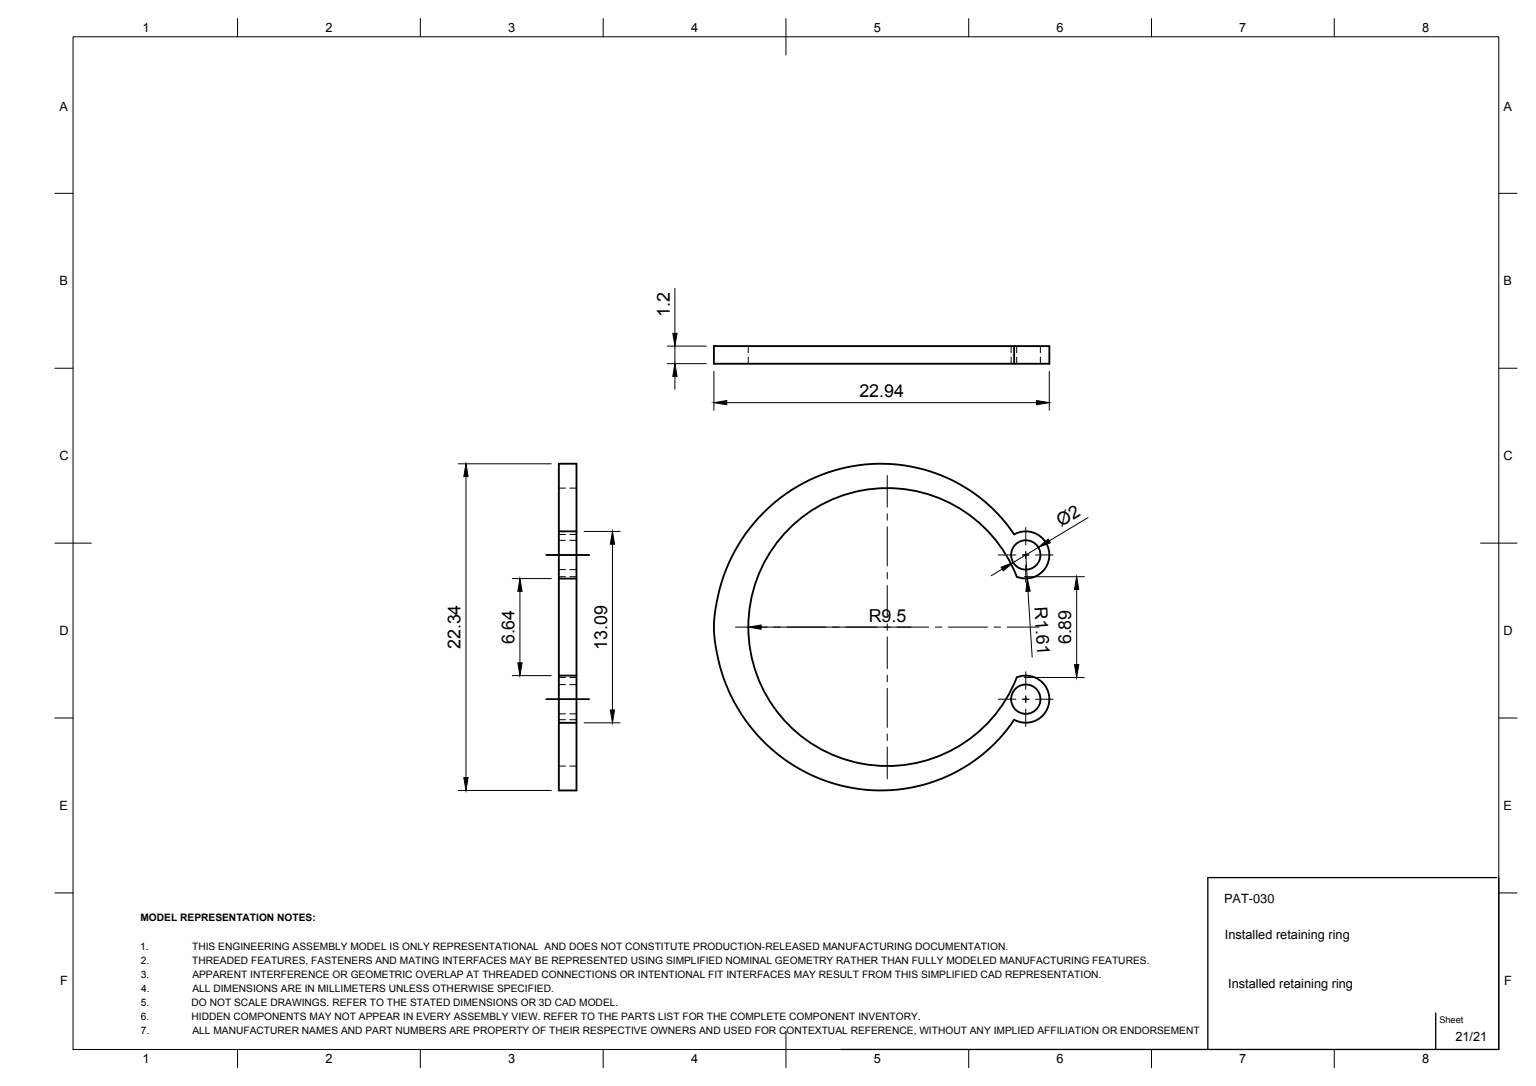
ISO-10303-21;
HEADER;
/* Generated by software containing ST-Developer
 * from STEP Tools, Inc. (www.steptools.com) 
 */

FILE_DESCRIPTION(
/* description */ ('Double-bearing flanged cartridge'),
/* implementation_level */ '2;1');

FILE_NAME(
/* name */ 'Installed retaining ring.step',
/* time_stamp */ '2026-10-28T03:26:40-07:00',
/* author */ (''),
/* organization */ (''),
/* preprocessor_version */ 'ST-DEVELOPER v20.2',
/* originating_system */ 'Autodesk Translation Framework v15.17.0.0',
/* authorisation */ '');

FILE_SCHEMA (('AUTOMOTIVE_DESIGN { 1 0 10303 214 3 1 1 }'));
ENDSEC;

DATA;
#10=MECHANICAL_DESIGN_GEOMETRIC_PRESENTATION_REPRESENTATION('',(#211),#5535);
#11=(
BOUNDED_SURFACE()
B_SPLINE_SURFACE(5,1,((#4887,#4888),(#4889,#4890),(#4891,#4892),(#4893,
#4894),(#4895,#4896),(#4897,#4898),(#4899,#4900),(#4901,#4902),(#4903,#4904),
(#4905,#4906),(#4907,#4908),(#4909,#4910),(#4911,#4912),(#4913,#4914),(#4915,
#4916),(#4917,#4918),(#4919,#4920),(#4921,#4922),(#4923,#4924),(#4925,#4926),
(#4927,#4928),(#4929,#4930),(#4931,#4932),(#4933,#4934),(#4935,#4936),(#4937,
#4938),(#4939,#4940),(#4941,#4942),(#4943,#4944),(#4945,#4946),(#4947,#4948),
(#4949,#4950),(#4951,#4952),(#4953,#4954),(#4955,#4956),(#4957,#4958),(#4959,
#4960),(#4961,#4962),(#4963,#4964),(#4965,#4966),(#4967,#4968),(#4969,#4970),
(#4971,#4972),(#4973,#4974),(#4975,#4976),(#4977,#4978),(#4979,#4980),(#4981,
#4982),(#4983,#4984),(#4985,#4986),(#4987,#4988),(#4989,#4990),(#4991,#4992),
(#4993,#4994),(#4995,#4996),(#4997,#4998),(#4999,#5000),(#5001,#5002),(#5003,
#5004),(#5005,#5006),(#5007,#5008),(#5009,#5010),(#5011,#5012),(#5013,#5014),
(#5015,#5016),(#5017,#5018),(#5019,#5020),(#5021,#5022),(#5023,#5024),(#5025,
#5026),(#5027,#5028),(#5029,#5030),(#5031,#5032),(#5033,#5034),(#5035,#5036),
(#5037,#5038),(#5039,#5040),(#5041,#5042),(#5043,#5044),(#5045,#5046),(#5047,
#5048),(#5049,#5050),(#5051,#5052),(#5053,#5054),(#5055,#5056),(#5057,#5058),
(#5059,#5060),(#5061,#5062),(#5063,#5064),(#5065,#5066),(#5067,#5068),(#5069,
#5070),(#5071,#5072),(#5073,#5074),(#5075,#5076),(#5077,#5078),(#5079,#5080),
(#5081,#5082),(#5083,#5084),(#5085,#5086),(#5087,#5088),(#5089,#5090),(#5091,
#5092),(#5093,#5094),(#5095,#5096),(#5097,#5098),(#5099,#5100),(#5101,#5102),
(#5103,#5104),(#5105,#5106),(#5107,#5108),(#5109,#5110),(#5111,#5112),(#5113,
#5114),(#5115,#5116),(#5117,#5118),(#5119,#5120),(#5121,#5122),(#5123,#5124),
(#5125,#5126),(#5127,#5128),(#5129,#5130),(#5131,#5132),(#5133,#5134),(#5135,
#5136),(#5137,#5138),(#5139,#5140),(#5141,#5142),(#5143,#5144),(#5145,#5146),
(#5147,#5148),(#5149,#5150),(#5151,#5152),(#5153,#5154),(#5155,#5156),(#5157,
#5158),(#5159,#5160),(#5161,#5162),(#5163,#5164),(#5165,#5166),(#5167,#5168),
(#5169,#5170),(#5171,#5172),(#5173,#5174),(#5175,#5176),(#5177,#5178),(#5179,
#5180),(#5181,#5182),(#5183,#5184),(#5185,#5186),(#5187,#5188),(#5189,#5190),
(#5191,#5192),(#5193,#5194),(#5195,#5196),(#5197,#5198),(#5199,#5200),(#5201,
#5202),(#5203,#5204),(#5205,#5206),(#5207,#5208),(#5209,#5210),(#5211,#5212),
(#5213,#5214),(#5215,#5216),(#5217,#5218),(#5219,#5220),(#5221,#5222),(#5223,
#5224),(#5225,#5226),(#5227,#5228),(#5229,#5230),(#5231,#5232),(#5233,#5234),
(#5235,#5236),(#5237,#5238),(#5239,#5240),(#5241,#5242),(#5243,#5244),(#5245,
#5246),(#5247,#5248),(#5249,#5250),(#5251,#5252),(#5253,#5254),(#5255,#5256),
(#5257,#5258),(#5259,#5260),(#5261,#5262),(#5263,#5264),(#5265,#5266),(#5267,
#5268),(#5269,#5270),(#5271,#5272),(#5273,#5274),(#5275,#5276),(#5277,#5278),
(#5279,#5280),(#5281,#5282),(#5283,#5284),(#5285,#5286),(#5287,#5288),(#5289,
#5290),(#5291,#5292),(#5293,#5294),(#5295,#5296)),.UNSPECIFIED.,.F.,.F.,
 .F.)
B_SPLINE_SURFACE_WITH_KNOTS((6,1,1,1,1,1,1,1,1,1,1,1,1,1,1,1,1,1,1,1,1,
1,1,1,1,1,1,1,1,1,1,1,1,1,1,1,1,1,1,1,1,1,1,1,1,1,1,1,1,1,1,1,1,1,1,1,1,
1,1,1,1,1,1,1,1,1,1,1,1,1,1,1,1,1,1,1,1,1,1,1,1,1,1,1,1,1,1,1,1,1,1,1,1,
1,1,1,1,1,1,1,1,1,1,1,1,1,1,1,1,1,1,1,1,1,1,1,1,1,1,1,1,1,1,1,1,1,1,1,1,
1,1,1,1,1,1,1,1,1,1,1,1,1,1,1,1,1,1,1,1,1,1,1,1,1,1,1,1,1,1,1,1,1,1,1,1,
1,1,1,1,1,1,1,1,1,1,1,1,1,1,1,1,1,1,1,1,1,1,1,1,1,1,1,1,1,1,1,1,1,1,1,6),
(2,2),(0.,0.005,0.01,0.015,0.02,0.025,0.03,0.035,0.04,0.045,0.05,0.055,
0.06,0.065,0.07,0.075,0.08,0.085,0.09,0.095,0.1,0.105,0.11,0.115,0.12,0.125,
0.13,0.135,0.14,0.145,0.15,0.155,0.16,0.165,0.17,0.175,0.18,0.185,0.19,
0.195,0.2,0.205,0.21,0.215,0.22,0.225,0.23,0.235,0.24,0.245,0.25,0.255,
0.26,0.265,0.27,0.275,0.28,0.285,0.29,0.295,0.3,0.305,0.31,0.315,0.32,0.325,
0.33,0.335,0.34,0.345,0.35,0.355,0.36,0.365,0.37,0.375,0.38,0.385,0.39,
0.395,0.4,0.405,0.41,0.415,0.42,0.425,0.43,0.435,0.44,0.445,0.45,0.455,
0.46,0.465,0.47,0.475,0.48,0.485,0.49,0.495,0.5,0.505,0.51,0.515,0.52,0.525,
0.53,0.535,0.54,0.545,0.55,0.555,0.56,0.565,0.57,0.575,0.58,0.585,0.59,
0.595,0.6,0.605,0.61,0.615,0.62,0.625,0.63,0.635,0.64,0.645,0.65,0.655,
0.66,0.665,0.67,0.675,0.68,0.685,0.690000000000001,0.695000000000001,0.700000000000001,
0.705000000000001,0.710000000000001,0.715000000000001,0.720000000000001,
0.725000000000001,0.730000000000001,0.735000000000001,0.740000000000001,
0.745000000000001,0.750000000000001,0.755000000000001,0.760000000000001,
0.765000000000001,0.770000000000001,0.775000000000001,0.780000000000001,
0.785000000000001,0.790000000000001,0.795000000000001,0.800000000000001,
0.805000000000001,0.810000000000001,0.815000000000001,0.820000000000001,
0.825000000000001,0.830000000000001,0.835000000000001,0.840000000000001,
0.845000000000001,0.850000000000001,0.855000000000001,0.860000000000001,
0.865000000000001,0.870000000000001,0.875000000000001,0.880000000000001,
0.885000000000001,0.890000000000001,0.895000000000001,0.900000000000001,
0.905000000000001,0.910000000000001,0.915000000000001,0.920000000000001,
0.925000000000001,0.930000000000001,0.935000000000001,0.940000000000001,
0.945000000000001,0.950000000000001,0.955000000000001,0.960000000000001,
0.965000000000001,0.970000000000001,0.975000000000001,0.980000000000001,
0.985000000000001,0.990000000000001,0.995000000000001,1.),(0.,0.12),
 .UNSPECIFIED.)
GEOMETRIC_REPRESENTATION_ITEM()
RATIONAL_B_SPLINE_SURFACE(((1.,1.),(1.,1.),(1.,1.),(1.,1.),(1.,1.),(1.,
1.),(1.,1.),(1.,1.),(1.,1.),(1.,1.),(1.,1.),(1.,1.),(1.,1.),(1.,1.),(1.,
1.),(1.,1.),(1.,1.),(1.,1.),(1.,1.),(1.,1.),(1.,1.),(1.,1.),(1.,1.),(1.,
1.),(1.,1.),(1.,1.),(1.,1.),(1.,1.),(1.,1.),(1.,1.),(1.,1.),(1.,1.),(1.,
1.),(1.,1.),(1.,1.),(1.,1.),(1.,1.),(1.,1.),(1.,1.),(1.,1.),(1.,1.),(1.,
1.),(1.,1.),(1.,1.),(1.,1.),(1.,1.),(1.,1.),(1.,1.),(1.,1.),(1.,1.),(1.,
1.),(1.,1.),(1.,1.),(1.,1.),(1.,1.),(1.,1.),(1.,1.),(1.,1.),(1.,1.),(1.,
1.),(1.,1.),(1.,1.),(1.,1.),(1.,1.),(1.,1.),(1.,1.),(1.,1.),(1.,1.),(1.,
1.),(1.,1.),(1.,1.),(1.,1.),(1.,1.),(1.,1.),(1.,1.),(1.,1.),(1.,1.),(1.,
1.),(1.,1.),(1.,1.),(1.,1.),(1.,1.),(1.,1.),(1.,1.),(1.,1.),(1.,1.),(1.,
1.),(1.,1.),(1.,1.),(1.,1.),(1.,1.),(1.,1.),(1.,1.),(1.,1.),(1.,1.),(1.,
1.),(1.,1.),(1.,1.),(1.,1.),(1.,1.),(1.,1.),(1.,1.),(1.,1.),(1.,1.),(1.,
1.),(1.,1.),(1.,1.),(1.,1.),(1.,1.),(1.,1.),(1.,1.),(1.,1.),(1.,1.),(1.,
1.),(1.,1.),(1.,1.),(1.,1.),(1.,1.),(1.,1.),(1.,1.),(1.,1.),(1.,1.),(1.,
1.),(1.,1.),(1.,1.),(1.,1.),(1.,1.),(1.,1.),(1.,1.),(1.,1.),(1.,1.),(1.,
1.),(1.,1.),(1.,1.),(1.,1.),(1.,1.),(1.,1.),(1.,1.),(1.,1.),(1.,1.),(1.,
1.),(1.,1.),(1.,1.),(1.,1.),(1.,1.),(1.,1.),(1.,1.),(1.,1.),(1.,1.),(1.,
1.),(1.,1.),(1.,1.),(1.,1.),(1.,1.),(1.,1.),(1.,1.),(1.,1.),(1.,1.),(1.,
1.),(1.,1.),(1.,1.),(1.,1.),(1.,1.),(1.,1.),(1.,1.),(1.,1.),(1.,1.),(1.,
1.),(1.,1.),(1.,1.),(1.,1.),(1.,1.),(1.,1.),(1.,1.),(1.,1.),(1.,1.),(1.,
1.),(1.,1.),(1.,1.),(1.,1.),(1.,1.),(1.,1.),(1.,1.),(1.,1.),(1.,1.),(1.,
1.),(1.,1.),(1.,1.),(1.,1.),(1.,1.),(1.,1.),(1.,1.),(1.,1.),(1.,1.),(1.,
1.),(1.,1.),(1.,1.),(1.,1.),(1.,1.),(1.,1.),(1.,1.),(1.,1.),(1.,1.),(1.,
1.),(1.,1.)))
REPRESENTATION_ITEM('')
SURFACE()
);
#12=(
BOUNDED_CURVE()
B_SPLINE_CURVE(5,(#4671,#4672,#4673,#4674,#4675,#4676,#4677,#4678,#4679,
#4680,#4681,#4682,#4683,#4684,#4685,#4686,#4687,#4688,#4689,#4690,#4691,
#4692,#4693,#4694,#4695,#4696,#4697,#4698,#4699,#4700,#4701,#4702,#4703,
#4704,#4705,#4706,#4707,#4708,#4709,#4710,#4711,#4712,#4713,#4714,#4715,
#4716,#4717,#4718,#4719,#4720,#4721,#4722,#4723,#4724,#4725,#4726,#4727,
#4728,#4729,#4730,#4731,#4732,#4733,#4734,#4735,#4736,#4737,#4738,#4739,
#4740,#4741,#4742,#4743,#4744,#4745,#4746,#4747,#4748,#4749,#4750,#4751,
#4752,#4753,#4754,#4755,#4756,#4757,#4758,#4759,#4760,#4761,#4762,#4763,
#4764,#4765,#4766,#4767,#4768,#4769,#4770,#4771,#4772,#4773,#4774,#4775,
#4776,#4777,#4778,#4779,#4780,#4781,#4782,#4783,#4784,#4785,#4786,#4787,
#4788,#4789,#4790,#4791,#4792,#4793,#4794,#4795,#4796,#4797,#4798,#4799,
#4800,#4801,#4802,#4803,#4804,#4805,#4806,#4807,#4808,#4809,#4810,#4811,
#4812,#4813,#4814,#4815,#4816,#4817,#4818,#4819,#4820,#4821,#4822,#4823,
#4824,#4825,#4826,#4827,#4828,#4829,#4830,#4831,#4832,#4833,#4834,#4835,
#4836,#4837,#4838,#4839,#4840,#4841,#4842,#4843,#4844,#4845,#4846,#4847,
#4848,#4849,#4850,#4851,#4852,#4853,#4854,#4855,#4856,#4857,#4858,#4859,
#4860,#4861,#4862,#4863,#4864,#4865),.UNSPECIFIED.,.F.,.F.)
B_SPLINE_CURVE_WITH_KNOTS((6,1,1,1,1,1,1,1,1,1,1,1,1,1,1,1,1,1,1,1,1,1,
1,1,1,1,1,1,1,1,1,1,1,1,1,1,1,1,1,1,1,1,1,1,1,1,1,1,1,1,1,1,1,1,1,1,1,1,
1,1,1,1,1,1,1,1,1,1,1,1,1,1,1,1,1,1,1,1,1,1,1,1,1,1,1,1,1,1,1,1,1,1,1,1,
1,1,1,1,1,1,1,1,1,1,1,1,1,1,1,1,1,1,1,1,1,1,1,1,1,1,1,1,1,1,1,1,1,1,1,1,
1,1,1,1,1,1,1,1,1,1,1,1,1,1,1,1,1,1,1,1,1,1,1,1,1,1,1,1,1,1,1,1,1,1,1,1,
1,1,1,1,1,1,1,1,1,1,1,1,1,1,1,1,1,1,1,1,1,1,1,1,6),(0.02759962388435,0.03,
0.035,0.04,0.045,0.05,0.055,0.06,0.065,0.07,0.075,0.08,0.085,0.09,0.095,
0.1,0.105,0.11,0.115,0.12,0.125,0.13,0.135,0.14,0.145,0.15,0.155,0.16,0.165,
0.17,0.175,0.18,0.185,0.19,0.195,0.2,0.205,0.21,0.215,0.22,0.225,0.23,0.235,
0.24,0.245,0.25,0.255,0.26,0.265,0.27,0.275,0.28,0.285,0.29,0.295,0.3,0.305,
0.31,0.315,0.32,0.325,0.33,0.335,0.34,0.345,0.35,0.355,0.36,0.365,0.37,
0.375,0.38,0.385,0.39,0.395,0.4,0.405,0.41,0.415,0.42,0.425,0.43,0.435,
0.44,0.445,0.45,0.455,0.46,0.465,0.47,0.475,0.48,0.485,0.49,0.495,0.5,0.505,
0.51,0.515,0.52,0.525,0.53,0.535,0.54,0.545,0.55,0.555,0.56,0.565,0.57,
0.575,0.58,0.585,0.59,0.595,0.6,0.605,0.61,0.615,0.62,0.625,0.63,0.635,
0.64,0.645,0.65,0.655,0.66,0.665,0.67,0.675,0.68,0.685,0.690000000000001,
0.695000000000001,0.700000000000001,0.705000000000001,0.710000000000001,
0.715000000000001,0.720000000000001,0.725000000000001,0.730000000000001,
0.735000000000001,0.740000000000001,0.745000000000001,0.750000000000001,
0.755000000000001,0.760000000000001,0.765000000000001,0.770000000000001,
0.775000000000001,0.780000000000001,0.785000000000001,0.790000000000001,
0.795000000000001,0.800000000000001,0.805000000000001,0.810000000000001,
0.815000000000001,0.820000000000001,0.825000000000001,0.830000000000001,
0.835000000000001,0.840000000000001,0.845000000000001,0.850000000000001,
0.855000000000001,0.860000000000001,0.865000000000001,0.870000000000001,
0.875000000000001,0.880000000000001,0.885000000000001,0.890000000000001,
0.895000000000001,0.900000000000001,0.905000000000001,0.910000000000001,
0.915000000000001,0.920000000000001,0.925000000000001,0.930000000000001,
0.935000000000001,0.940000000000001,0.945000000000001,0.950000000000001,
0.955000000000001,0.960000000000001,0.965000000000001,0.970000000000001,
0.972400376115677),.UNSPECIFIED.)
CURVE()
GEOMETRIC_REPRESENTATION_ITEM()
RATIONAL_B_SPLINE_CURVE((1.,1.,1.,1.,1.,1.,1.,1.,1.,1.,1.,1.,1.,1.,1.,1.,
1.,1.,1.,1.,1.,1.,1.,1.,1.,1.,1.,1.,1.,1.,1.,1.,1.,1.,1.,1.,1.,1.,1.,1.,
1.,1.,1.,1.,1.,1.,1.,1.,1.,1.,1.,1.,1.,1.,1.,1.,1.,1.,1.,1.,1.,1.,1.,1.,
1.,1.,1.,1.,1.,1.,1.,1.,1.,1.,1.,1.,1.,1.,1.,1.,1.,1.,1.,1.,1.,1.,1.,1.,
1.,1.,1.,1.,1.,1.,1.,1.,1.,1.,1.,1.,1.,1.,1.,1.,1.,1.,1.,1.,1.,1.,1.,1.,
1.,1.,1.,1.,1.,1.,1.,1.,1.,1.,1.,1.,1.,1.,1.,1.,1.,1.,1.,1.,1.,1.,1.,1.,
1.,1.,1.,1.,1.,1.,1.,1.,1.,1.,1.,1.,1.,1.,1.,1.,1.,1.,1.,1.,1.,1.,1.,1.,
1.,1.,1.,1.,1.,1.,1.,1.,1.,1.,1.,1.,1.,1.,1.,1.,1.,1.,1.,1.,1.,1.,1.,1.,
1.,1.,1.,1.,1.,1.,1.,1.,1.,1.,1.))
REPRESENTATION_ITEM('')
);
#13=(
BOUNDED_CURVE()
B_SPLINE_CURVE(5,(#5297,#5298,#5299,#5300,#5301,#5302,#5303,#5304,#5305,
#5306,#5307,#5308,#5309,#5310,#5311,#5312,#5313,#5314,#5315,#5316,#5317,
#5318,#5319,#5320,#5321,#5322,#5323,#5324,#5325,#5326,#5327,#5328,#5329,
#5330,#5331,#5332,#5333,#5334,#5335,#5336,#5337,#5338,#5339,#5340,#5341,
#5342,#5343,#5344,#5345,#5346,#5347,#5348,#5349,#5350,#5351,#5352,#5353,
#5354,#5355,#5356,#5357,#5358,#5359,#5360,#5361,#5362,#5363,#5364,#5365,
#5366,#5367,#5368,#5369,#5370,#5371,#5372,#5373,#5374,#5375,#5376,#5377,
#5378,#5379,#5380,#5381,#5382,#5383,#5384,#5385,#5386,#5387,#5388,#5389,
#5390,#5391,#5392,#5393,#5394,#5395,#5396,#5397,#5398,#5399,#5400,#5401,
#5402,#5403,#5404,#5405,#5406,#5407,#5408,#5409,#5410,#5411,#5412,#5413,
#5414,#5415,#5416,#5417,#5418,#5419,#5420,#5421,#5422,#5423,#5424,#5425,
#5426,#5427,#5428,#5429,#5430,#5431,#5432,#5433,#5434,#5435,#5436,#5437,
#5438,#5439,#5440,#5441,#5442,#5443,#5444,#5445,#5446,#5447,#5448,#5449,
#5450,#5451,#5452,#5453,#5454,#5455,#5456,#5457,#5458,#5459,#5460,#5461,
#5462,#5463,#5464,#5465,#5466,#5467,#5468,#5469,#5470,#5471,#5472,#5473,
#5474,#5475,#5476,#5477,#5478,#5479,#5480,#5481,#5482,#5483,#5484,#5485,
#5486,#5487,#5488,#5489,#5490,#5491),.UNSPECIFIED.,.F.,.F.)
B_SPLINE_CURVE_WITH_KNOTS((6,1,1,1,1,1,1,1,1,1,1,1,1,1,1,1,1,1,1,1,1,1,
1,1,1,1,1,1,1,1,1,1,1,1,1,1,1,1,1,1,1,1,1,1,1,1,1,1,1,1,1,1,1,1,1,1,1,1,
1,1,1,1,1,1,1,1,1,1,1,1,1,1,1,1,1,1,1,1,1,1,1,1,1,1,1,1,1,1,1,1,1,1,1,1,
1,1,1,1,1,1,1,1,1,1,1,1,1,1,1,1,1,1,1,1,1,1,1,1,1,1,1,1,1,1,1,1,1,1,1,1,
1,1,1,1,1,1,1,1,1,1,1,1,1,1,1,1,1,1,1,1,1,1,1,1,1,1,1,1,1,1,1,1,1,1,1,1,
1,1,1,1,1,1,1,1,1,1,1,1,1,1,1,1,1,1,1,1,1,1,1,1,6),(0.02759962388435,0.03,
0.035,0.04,0.045,0.05,0.055,0.06,0.065,0.07,0.075,0.08,0.085,0.09,0.095,
0.1,0.105,0.11,0.115,0.12,0.125,0.13,0.135,0.14,0.145,0.15,0.155,0.16,0.165,
0.17,0.175,0.18,0.185,0.19,0.195,0.2,0.205,0.21,0.215,0.22,0.225,0.23,0.235,
0.24,0.245,0.25,0.255,0.26,0.265,0.27,0.275,0.28,0.285,0.29,0.295,0.3,0.305,
0.31,0.315,0.32,0.325,0.33,0.335,0.34,0.345,0.35,0.355,0.36,0.365,0.37,
0.375,0.38,0.385,0.39,0.395,0.4,0.405,0.41,0.415,0.42,0.425,0.43,0.435,
0.44,0.445,0.45,0.455,0.46,0.465,0.47,0.475,0.48,0.485,0.49,0.495,0.5,0.505,
0.51,0.515,0.52,0.525,0.53,0.535,0.54,0.545,0.55,0.555,0.56,0.565,0.57,
0.575,0.58,0.585,0.59,0.595,0.6,0.605,0.61,0.615,0.62,0.625,0.63,0.635,
0.64,0.645,0.65,0.655,0.66,0.665,0.67,0.675,0.68,0.685,0.690000000000001,
0.695000000000001,0.700000000000001,0.705000000000001,0.710000000000001,
0.715000000000001,0.720000000000001,0.725000000000001,0.730000000000001,
0.735000000000001,0.740000000000001,0.745000000000001,0.750000000000001,
0.755000000000001,0.760000000000001,0.765000000000001,0.770000000000001,
0.775000000000001,0.780000000000001,0.785000000000001,0.790000000000001,
0.795000000000001,0.800000000000001,0.805000000000001,0.810000000000001,
0.815000000000001,0.820000000000001,0.825000000000001,0.830000000000001,
0.835000000000001,0.840000000000001,0.845000000000001,0.850000000000001,
0.855000000000001,0.860000000000001,0.865000000000001,0.870000000000001,
0.875000000000001,0.880000000000001,0.885000000000001,0.890000000000001,
0.895000000000001,0.900000000000001,0.905000000000001,0.910000000000001,
0.915000000000001,0.920000000000001,0.925000000000001,0.930000000000001,
0.935000000000001,0.940000000000001,0.945000000000001,0.950000000000001,
0.955000000000001,0.960000000000001,0.965000000000001,0.970000000000001,
0.972400376115677),.UNSPECIFIED.)
CURVE()
GEOMETRIC_REPRESENTATION_ITEM()
RATIONAL_B_SPLINE_CURVE((1.,1.,1.,1.,1.,1.,1.,1.,1.,1.,1.,1.,1.,1.,1.,1.,
1.,1.,1.,1.,1.,1.,1.,1.,1.,1.,1.,1.,1.,1.,1.,1.,1.,1.,1.,1.,1.,1.,1.,1.,
1.,1.,1.,1.,1.,1.,1.,1.,1.,1.,1.,1.,1.,1.,1.,1.,1.,1.,1.,1.,1.,1.,1.,1.,
1.,1.,1.,1.,1.,1.,1.,1.,1.,1.,1.,1.,1.,1.,1.,1.,1.,1.,1.,1.,1.,1.,1.,1.,
1.,1.,1.,1.,1.,1.,1.,1.,1.,1.,1.,1.,1.,1.,1.,1.,1.,1.,1.,1.,1.,1.,1.,1.,
1.,1.,1.,1.,1.,1.,1.,1.,1.,1.,1.,1.,1.,1.,1.,1.,1.,1.,1.,1.,1.,1.,1.,1.,
1.,1.,1.,1.,1.,1.,1.,1.,1.,1.,1.,1.,1.,1.,1.,1.,1.,1.,1.,1.,1.,1.,1.,1.,
1.,1.,1.,1.,1.,1.,1.,1.,1.,1.,1.,1.,1.,1.,1.,1.,1.,1.,1.,1.,1.,1.,1.,1.,
1.,1.,1.,1.,1.,1.,1.,1.,1.,1.,1.))
REPRESENTATION_ITEM('')
);
#134=B_SPLINE_CURVE_WITH_KNOTS('',3,(#4661,#4662,#4663,#4664,#4665,#4666),
 .UNSPECIFIED.,.F.,.F.,(4,2,4),(-0.12,-0.06,0.),.UNSPECIFIED.);
#135=B_SPLINE_CURVE_WITH_KNOTS('',3,(#4881,#4882,#4883,#4884,#4885,#4886),
 .UNSPECIFIED.,.F.,.F.,(4,2,4),(-0.12,-0.06,0.),.UNSPECIFIED.);
#175=SHAPE_REPRESENTATION_RELATIONSHIP('SRR','None',#5618,#189);
#189=ADVANCED_BREP_SHAPE_REPRESENTATION('',(#232),#5534);
#211=STYLED_ITEM('',(#5778),#232);
#232=MANIFOLD_SOLID_BREP('Body1',#2346);
#296=FACE_BOUND('',#717,.T.);
#297=FACE_BOUND('',#718,.T.);
#298=FACE_BOUND('',#724,.T.);
#299=FACE_BOUND('',#725,.T.);
#359=PLANE('',#2851);
#360=PLANE('',#2861);
#502=FACE_OUTER_BOUND('',#714,.T.);
#503=FACE_OUTER_BOUND('',#715,.T.);
#504=FACE_OUTER_BOUND('',#716,.T.);
#505=FACE_OUTER_BOUND('',#719,.T.);
#506=FACE_OUTER_BOUND('',#720,.T.);
#507=FACE_OUTER_BOUND('',#721,.T.);
#508=FACE_OUTER_BOUND('',#722,.T.);
#509=FACE_OUTER_BOUND('',#723,.T.);
#714=EDGE_LOOP('',(#2078,#2079,#2080,#2081));
#715=EDGE_LOOP('',(#2082,#2083,#2084,#2085));
#716=EDGE_LOOP('',(#2086,#2087,#2088,#2089));
#717=EDGE_LOOP('',(#2090));
#718=EDGE_LOOP('',(#2091));
#719=EDGE_LOOP('',(#2092,#2093,#2094,#2095));
#720=EDGE_LOOP('',(#2096,#2097,#2098,#2099));
#721=EDGE_LOOP('',(#2100,#2101,#2102,#2103));
#722=EDGE_LOOP('',(#2104,#2105,#2106,#2107));
#723=EDGE_LOOP('',(#2108,#2109,#2110,#2111));
#724=EDGE_LOOP('',(#2112));
#725=EDGE_LOOP('',(#2113));
#808=LINE('',#4651,#894);
#809=LINE('',#4655,#895);
#810=LINE('',#4872,#896);
#811=LINE('',#4876,#897);
#894=VECTOR('',#3637,1.);
#895=VECTOR('',#3640,1.);
#896=VECTOR('',#3659,0.1);
#897=VECTOR('',#3664,0.1);
#1062=CIRCLE('',#2846,0.95);
#1063=CIRCLE('',#2847,0.95);
#1064=CIRCLE('',#2849,0.1612);
#1065=CIRCLE('',#2850,0.1612);
#1066=CIRCLE('',#2852,0.1612);
#1067=CIRCLE('',#2853,0.1);
#1068=CIRCLE('',#2854,0.1);
#1069=CIRCLE('',#2856,0.1);
#1070=CIRCLE('',#2858,0.1);
#1071=CIRCLE('',#2860,0.1612);
#1256=VERTEX_POINT('',#4649);
#1257=VERTEX_POINT('',#4650);
#1258=VERTEX_POINT('',#4652);
#1259=VERTEX_POINT('',#4654);
#1260=VERTEX_POINT('',#4658);
#1261=VERTEX_POINT('',#4660);
#1262=VERTEX_POINT('',#4669);
#1263=VERTEX_POINT('',#4866);
#1264=VERTEX_POINT('',#4868);
#1265=VERTEX_POINT('',#4871);
#1266=VERTEX_POINT('',#4875);
#1267=VERTEX_POINT('',#4879);
#1532=EDGE_CURVE('',#1256,#1257,#808,.T.);
#1533=EDGE_CURVE('',#1258,#1256,#1062,.T.);
#1534=EDGE_CURVE('',#1259,#1258,#809,.T.);
#1535=EDGE_CURVE('',#1257,#1259,#1063,.T.);
#1536=EDGE_CURVE('',#1258,#1260,#1064,.T.);
#1537=EDGE_CURVE('',#1261,#1260,#134,.T.);
#1538=EDGE_CURVE('',#1259,#1261,#1065,.T.);
#1539=EDGE_CURVE('',#1262,#1256,#1066,.T.);
#1540=EDGE_CURVE('',#1260,#1262,#12,.T.);
#1541=EDGE_CURVE('',#1263,#1263,#1067,.T.);
#1542=EDGE_CURVE('',#1264,#1264,#1068,.T.);
#1543=EDGE_CURVE('',#1264,#1265,#810,.T.);
#1544=EDGE_CURVE('',#1265,#1265,#1069,.T.);
#1545=EDGE_CURVE('',#1263,#1266,#811,.T.);
#1546=EDGE_CURVE('',#1266,#1266,#1070,.T.);
#1547=EDGE_CURVE('',#1267,#1257,#1071,.T.);
#1548=EDGE_CURVE('',#1262,#1267,#135,.T.);
#1549=EDGE_CURVE('',#1261,#1267,#13,.T.);
#2078=ORIENTED_EDGE('',*,*,#1532,.F.);
#2079=ORIENTED_EDGE('',*,*,#1533,.F.);
#2080=ORIENTED_EDGE('',*,*,#1534,.F.);
#2081=ORIENTED_EDGE('',*,*,#1535,.F.);
#2082=ORIENTED_EDGE('',*,*,#1534,.T.);
#2083=ORIENTED_EDGE('',*,*,#1536,.T.);
#2084=ORIENTED_EDGE('',*,*,#1537,.F.);
#2085=ORIENTED_EDGE('',*,*,#1538,.F.);
#2086=ORIENTED_EDGE('',*,*,#1533,.T.);
#2087=ORIENTED_EDGE('',*,*,#1539,.F.);
#2088=ORIENTED_EDGE('',*,*,#1540,.F.);
#2089=ORIENTED_EDGE('',*,*,#1536,.F.);
#2090=ORIENTED_EDGE('',*,*,#1541,.T.);
#2091=ORIENTED_EDGE('',*,*,#1542,.T.);
#2092=ORIENTED_EDGE('',*,*,#1542,.F.);
#2093=ORIENTED_EDGE('',*,*,#1543,.T.);
#2094=ORIENTED_EDGE('',*,*,#1544,.F.);
#2095=ORIENTED_EDGE('',*,*,#1543,.F.);
#2096=ORIENTED_EDGE('',*,*,#1541,.F.);
#2097=ORIENTED_EDGE('',*,*,#1545,.T.);
#2098=ORIENTED_EDGE('',*,*,#1546,.F.);
#2099=ORIENTED_EDGE('',*,*,#1545,.F.);
#2100=ORIENTED_EDGE('',*,*,#1532,.T.);
#2101=ORIENTED_EDGE('',*,*,#1547,.F.);
#2102=ORIENTED_EDGE('',*,*,#1548,.F.);
#2103=ORIENTED_EDGE('',*,*,#1539,.T.);
#2104=ORIENTED_EDGE('',*,*,#1548,.T.);
#2105=ORIENTED_EDGE('',*,*,#1549,.F.);
#2106=ORIENTED_EDGE('',*,*,#1537,.T.);
#2107=ORIENTED_EDGE('',*,*,#1540,.T.);
#2108=ORIENTED_EDGE('',*,*,#1535,.T.);
#2109=ORIENTED_EDGE('',*,*,#1538,.T.);
#2110=ORIENTED_EDGE('',*,*,#1549,.T.);
#2111=ORIENTED_EDGE('',*,*,#1547,.T.);
#2112=ORIENTED_EDGE('',*,*,#1544,.T.);
#2113=ORIENTED_EDGE('',*,*,#1546,.T.);
#2170=CYLINDRICAL_SURFACE('',#2845,0.95);
#2171=CYLINDRICAL_SURFACE('',#2848,0.1612);
#2172=CYLINDRICAL_SURFACE('',#2855,0.1);
#2173=CYLINDRICAL_SURFACE('',#2857,0.1);
#2174=CYLINDRICAL_SURFACE('',#2859,0.1612);
#2316=ADVANCED_FACE('',(#502),#2170,.F.);
#2317=ADVANCED_FACE('',(#503),#2171,.T.);
#2318=ADVANCED_FACE('',(#504,#296,#297),#359,.F.);
#2319=ADVANCED_FACE('',(#505),#2172,.F.);
#2320=ADVANCED_FACE('',(#506),#2173,.F.);
#2321=ADVANCED_FACE('',(#507),#2174,.T.);
#2322=ADVANCED_FACE('',(#508),#11,.T.);
#2323=ADVANCED_FACE('',(#509,#298,#299),#360,.T.);
#2346=CLOSED_SHELL('',(#2316,#2317,#2318,#2319,#2320,#2321,#2322,#2323));
#2844=AXIS2_PLACEMENT_3D('',#4647,#3633,#3634);
#2845=AXIS2_PLACEMENT_3D('',#4648,#3635,#3636);
#2846=AXIS2_PLACEMENT_3D('',#4653,#3638,#3639);
#2847=AXIS2_PLACEMENT_3D('',#4656,#3641,#3642);
#2848=AXIS2_PLACEMENT_3D('',#4657,#3643,#3644);
#2849=AXIS2_PLACEMENT_3D('',#4659,#3645,#3646);
#2850=AXIS2_PLACEMENT_3D('',#4667,#3647,#3648);
#2851=AXIS2_PLACEMENT_3D('',#4668,#3649,#3650);
#2852=AXIS2_PLACEMENT_3D('',#4670,#3651,#3652);
#2853=AXIS2_PLACEMENT_3D('',#4867,#3653,#3654);
#2854=AXIS2_PLACEMENT_3D('',#4869,#3655,#3656);
#2855=AXIS2_PLACEMENT_3D('',#4870,#3657,#3658);
#2856=AXIS2_PLACEMENT_3D('',#4873,#3660,#3661);
#2857=AXIS2_PLACEMENT_3D('',#4874,#3662,#3663);
#2858=AXIS2_PLACEMENT_3D('',#4877,#3665,#3666);
#2859=AXIS2_PLACEMENT_3D('',#4878,#3667,#3668);
#2860=AXIS2_PLACEMENT_3D('',#4880,#3669,#3670);
#2861=AXIS2_PLACEMENT_3D('',#5492,#3671,#3672);
#3633=DIRECTION('axis',(0.,0.,1.));
#3634=DIRECTION('refdir',(1.,0.,0.));
#3635=DIRECTION('center_axis',(0.,0.,1.));
#3636=DIRECTION('ref_axis',(1.,0.,0.));
#3637=DIRECTION('',(0.,0.,1.));
#3638=DIRECTION('center_axis',(0.,0.,1.));
#3639=DIRECTION('ref_axis',(1.,0.,0.));
#3640=DIRECTION('',(0.,0.,-1.));
#3641=DIRECTION('center_axis',(0.,0.,-1.));
#3642=DIRECTION('ref_axis',(1.,0.,0.));
#3643=DIRECTION('center_axis',(0.,0.,1.));
#3644=DIRECTION('ref_axis',(-0.998199433392819,-0.0599824238777901,0.));
#3645=DIRECTION('center_axis',(0.,0.,1.));
#3646=DIRECTION('ref_axis',(1.,0.,0.));
#3647=DIRECTION('center_axis',(0.,0.,1.));
#3648=DIRECTION('ref_axis',(1.,0.,0.));
#3649=DIRECTION('center_axis',(0.,0.,1.));
#3650=DIRECTION('ref_axis',(1.,0.,0.));
#3651=DIRECTION('center_axis',(0.,0.,1.));
#3652=DIRECTION('ref_axis',(1.,0.,0.));
#3653=DIRECTION('center_axis',(0.,0.,1.));
#3654=DIRECTION('ref_axis',(1.,0.,0.));
#3655=DIRECTION('center_axis',(0.,0.,1.));
#3656=DIRECTION('ref_axis',(1.,0.,0.));
#3657=DIRECTION('center_axis',(0.,0.,1.));
#3658=DIRECTION('ref_axis',(1.,0.,0.));
#3659=DIRECTION('',(0.,0.,1.));
#3660=DIRECTION('center_axis',(0.,0.,-1.));
#3661=DIRECTION('ref_axis',(1.,0.,0.));
#3662=DIRECTION('center_axis',(0.,0.,1.));
#3663=DIRECTION('ref_axis',(1.,0.,0.));
#3664=DIRECTION('',(0.,0.,1.));
#3665=DIRECTION('center_axis',(0.,0.,-1.));
#3666=DIRECTION('ref_axis',(1.,0.,0.));
#3667=DIRECTION('center_axis',(0.,0.,1.));
#3668=DIRECTION('ref_axis',(-0.998199433392758,0.0599824238788159,0.));
#3669=DIRECTION('center_axis',(0.,0.,1.));
#3670=DIRECTION('ref_axis',(1.,0.,0.));
#3671=DIRECTION('center_axis',(0.,0.,1.));
#3672=DIRECTION('ref_axis',(1.,0.,0.));
#4647=CARTESIAN_POINT('',(0.,0.,0.));
#4648=CARTESIAN_POINT('Origin',(0.,0.,-0.1));
#4649=CARTESIAN_POINT('',(-0.885408350996075,0.344313885846057,0.));
#4650=CARTESIAN_POINT('',(-0.885408350996075,0.344313885846057,0.12));
#4651=CARTESIAN_POINT('',(-0.885408350996075,0.344313885846057,-0.1));
#4652=CARTESIAN_POINT('',(-0.885408350996075,-0.344313885846057,0.));
#4653=CARTESIAN_POINT('Origin',(0.,0.,0.));
#4654=CARTESIAN_POINT('',(-0.885408350996075,-0.344313885846057,0.12));
#4655=CARTESIAN_POINT('',(-0.885408350996075,-0.344313885846057,-0.1));
#4656=CARTESIAN_POINT('Origin',(0.,0.,0.12));
#4657=CARTESIAN_POINT('Origin',(-0.947327569834341,-0.493147518935016,0.));
#4658=CARTESIAN_POINT('',(-0.8680312528477,-0.633495422775274,0.));
#4659=CARTESIAN_POINT('Origin',(-0.947327569834341,-0.493147518935016,0.));
#4660=CARTESIAN_POINT('',(-0.8680312528477,-0.633495422775274,0.12));
#4661=CARTESIAN_POINT('Ctrl Pts',(-0.8680312528477,-0.633495422775274,0.12));
#4662=CARTESIAN_POINT('Ctrl Pts',(-0.8680312528477,-0.633495422775274,0.1));
#4663=CARTESIAN_POINT('Ctrl Pts',(-0.8680312528477,-0.633495422775274,0.08));
#4664=CARTESIAN_POINT('Ctrl Pts',(-0.8680312528477,-0.633495422775274,0.04));
#4665=CARTESIAN_POINT('Ctrl Pts',(-0.8680312528477,-0.633495422775274,0.02));
#4666=CARTESIAN_POINT('Ctrl Pts',(-0.8680312528477,-0.633495422775274,0.));
#4667=CARTESIAN_POINT('Origin',(-0.947327569834341,-0.493147518935016,0.12));
#4668=CARTESIAN_POINT('Origin',(0.11901961308292,6.21724893790088E-15,0.));
#4669=CARTESIAN_POINT('',(-0.868031252847412,0.633495422775111,0.));
#4670=CARTESIAN_POINT('Origin',(-0.947327569834341,0.493147518935016,0.));
#4671=CARTESIAN_POINT('Ctrl Pts',(-0.8680312528477,-0.633495422775274,0.));
#4672=CARTESIAN_POINT('Ctrl Pts',(-0.866468860926997,-0.635830722731769,
0.));
#4673=CARTESIAN_POINT('Ctrl Pts',(-0.861627881960007,-0.64301558066062,
0.));
#4674=CARTESIAN_POINT('Ctrl Pts',(-0.853391883864834,-0.654977418032855,
0.));
#4675=CARTESIAN_POINT('Ctrl Pts',(-0.841545334406876,-0.671576597784011,
0.));
#4676=CARTESIAN_POINT('Ctrl Pts',(-0.82578008117756,-0.69259659895799,0.));
#4677=CARTESIAN_POINT('Ctrl Pts',(-0.807540237001814,-0.715586030006588,
0.));
#4678=CARTESIAN_POINT('Ctrl Pts',(-0.788671222413511,-0.738083066750504,
0.));
#4679=CARTESIAN_POINT('Ctrl Pts',(-0.769188516988648,-0.760067206050057,
0.));
#4680=CARTESIAN_POINT('Ctrl Pts',(-0.749106566399864,-0.781521126617586,
0.));
#4681=CARTESIAN_POINT('Ctrl Pts',(-0.728439343631846,-0.802429621210541,
0.));
#4682=CARTESIAN_POINT('Ctrl Pts',(-0.707200722570354,-0.822778881439107,
0.));
#4683=CARTESIAN_POINT('Ctrl Pts',(-0.685404899341998,-0.84255569314248,
0.));
#4684=CARTESIAN_POINT('Ctrl Pts',(-0.663066855029994,-0.861746554484541,
0.));
#4685=CARTESIAN_POINT('Ctrl Pts',(-0.640202597886525,-0.880337207900968,
0.));
#4686=CARTESIAN_POINT('Ctrl Pts',(-0.61682888916888,-0.898313140761512,
0.));
#4687=CARTESIAN_POINT('Ctrl Pts',(-0.592963069825771,-0.915659897318245,
0.));
#4688=CARTESIAN_POINT('Ctrl Pts',(-0.568622860345861,-0.932363440835334,
0.));
#4689=CARTESIAN_POINT('Ctrl Pts',(-0.543826140229843,-0.948410555212658,
0.));
#4690=CARTESIAN_POINT('Ctrl Pts',(-0.518590849350175,-0.963789014835703,
0.));
#4691=CARTESIAN_POINT('Ctrl Pts',(-0.492935086995462,-0.978487378620622,
0.));
#4692=CARTESIAN_POINT('Ctrl Pts',(-0.466877166338143,-0.992494869297879,
0.));
#4693=CARTESIAN_POINT('Ctrl Pts',(-0.440435680606148,-1.00580123015714,
0.));
#4694=CARTESIAN_POINT('Ctrl Pts',(-0.413629579915119,-1.01839656305955,
0.));
#4695=CARTESIAN_POINT('Ctrl Pts',(-0.386478184359591,-1.03027128325725,
0.));
#4696=CARTESIAN_POINT('Ctrl Pts',(-0.359001120477101,-1.04141621492846,
0.));
#4697=CARTESIAN_POINT('Ctrl Pts',(-0.331218276777395,-1.05182265203972,
0.));
#4698=CARTESIAN_POINT('Ctrl Pts',(-0.30314975447047,-1.06148242804708,0.));
#4699=CARTESIAN_POINT('Ctrl Pts',(-0.2748158132226,-1.07038799540312,0.));
#4700=CARTESIAN_POINT('Ctrl Pts',(-0.246236848114779,-1.07853244619974,
0.));
#4701=CARTESIAN_POINT('Ctrl Pts',(-0.217433396017985,-1.08590947721852,
0.));
#4702=CARTESIAN_POINT('Ctrl Pts',(-0.188426134393584,-1.09251336987768,
0.));
#4703=CARTESIAN_POINT('Ctrl Pts',(-0.159235881741527,-1.09833896639077,
0.));
#4704=CARTESIAN_POINT('Ctrl Pts',(-0.129883601129733,-1.10338164243564,
0.));
#4705=CARTESIAN_POINT('Ctrl Pts',(-0.100390386189668,-1.1076373045706,0.));
#4706=CARTESIAN_POINT('Ctrl Pts',(-0.0707774336926613,-1.11110240713062,
0.));
#4707=CARTESIAN_POINT('Ctrl Pts',(-0.0410660195909007,-1.11377396404697,
0.));
#4708=CARTESIAN_POINT('Ctrl Pts',(-0.0112774747954127,-1.11564956182599,
0.));
#4709=CARTESIAN_POINT('Ctrl Pts',(0.0185668417359402,-1.11672737500119,
0.));
#4710=CARTESIAN_POINT('Ctrl Pts',(0.0484455558693415,-1.11700616793207,
0.));
#4711=CARTESIAN_POINT('Ctrl Pts',(0.0783372821756426,-1.11648528736655,
0.));
#4712=CARTESIAN_POINT('Ctrl Pts',(0.108220629786098,-1.11516465787405,0.));
#4713=CARTESIAN_POINT('Ctrl Pts',(0.138074209040328,-1.1130447764894,0.));
#4714=CARTESIAN_POINT('Ctrl Pts',(0.167876633777266,-1.11012670736124,0.));
#4715=CARTESIAN_POINT('Ctrl Pts',(0.197606544321918,-1.10641207905813,0.));
#4716=CARTESIAN_POINT('Ctrl Pts',(0.227242642150327,-1.10190308368776,0.));
#4717=CARTESIAN_POINT('Ctrl Pts',(0.256763722532457,-1.09660247571268,0.));
#4718=CARTESIAN_POINT('Ctrl Pts',(0.286148704656023,-1.09051357088032,0.));
#4719=CARTESIAN_POINT('Ctrl Pts',(0.315376671295726,-1.08364024578391,0.));
#4720=CARTESIAN_POINT('Ctrl Pts',(0.344426864523868,-1.07598693493533,0.));
#4721=CARTESIAN_POINT('Ctrl Pts',(0.373278657560889,-1.06755862629372,0.));
#4722=CARTESIAN_POINT('Ctrl Pts',(0.40191153059007,-1.05836085760139,0.));
#4723=CARTESIAN_POINT('Ctrl Pts',(0.430305052465067,-1.04839971220046,0.));
#4724=CARTESIAN_POINT('Ctrl Pts',(0.45843884125875,-1.03768181616585,0.));
#4725=CARTESIAN_POINT('Ctrl Pts',(0.486292621102405,-1.02621433076827,0.));
#4726=CARTESIAN_POINT('Ctrl Pts',(0.513846332693361,-1.01400494236352,0.));
#4727=CARTESIAN_POINT('Ctrl Pts',(0.541080235433912,-1.00106185298107,0.));
#4728=CARTESIAN_POINT('Ctrl Pts',(0.567974995595113,-0.987393771329312,
0.));
#4729=CARTESIAN_POINT('Ctrl Pts',(0.594511824092215,-0.973009902467593,
0.));
#4730=CARTESIAN_POINT('Ctrl Pts',(0.620672396673315,-0.957919944163756,
0.));
#4731=CARTESIAN_POINT('Ctrl Pts',(0.646438641619482,-0.942134087249009,
0.));
#4732=CARTESIAN_POINT('Ctrl Pts',(0.67179254905522,-0.925663015702513,0.));
#4733=CARTESIAN_POINT('Ctrl Pts',(0.696716011515847,-0.908517905290565,
0.));
#4734=CARTESIAN_POINT('Ctrl Pts',(0.721190552023322,-0.890710427237186,
0.));
#4735=CARTESIAN_POINT('Ctrl Pts',(0.745197525414791,-0.872252731655685,
0.));
#4736=CARTESIAN_POINT('Ctrl Pts',(0.768718652031186,-0.853157416735685,
0.));
#4737=CARTESIAN_POINT('Ctrl Pts',(0.791736496209353,-0.833437500599933,
0.));
#4738=CARTESIAN_POINT('Ctrl Pts',(0.814234876393174,-0.81310639575503,0.));
#4739=CARTESIAN_POINT('Ctrl Pts',(0.836199528793963,-0.792177873864096,
0.));
#4740=CARTESIAN_POINT('Ctrl Pts',(0.857617760934752,-0.770666069833932,
0.));
#4741=CARTESIAN_POINT('Ctrl Pts',(0.878477242115376,-0.74858551944097,0.));
#4742=CARTESIAN_POINT('Ctrl Pts',(0.898764943113291,-0.725951191437368,
0.));
#4743=CARTESIAN_POINT('Ctrl Pts',(0.918466214618678,-0.70277851394702,0.));
#4744=CARTESIAN_POINT('Ctrl Pts',(0.937563319582499,-0.679083423181946,
0.));
#4745=CARTESIAN_POINT('Ctrl Pts',(0.956036026761672,-0.654882328595489,
0.));
#4746=CARTESIAN_POINT('Ctrl Pts',(0.973864462863685,-0.630191986422907,
0.));
#4747=CARTESIAN_POINT('Ctrl Pts',(0.991031566790864,-0.605029389584474,
0.));
#4748=CARTESIAN_POINT('Ctrl Pts',(1.00752529081786,-0.579411667627393,0.));
#4749=CARTESIAN_POINT('Ctrl Pts',(1.02334191285221,-0.553355942423953,0.));
#4750=CARTESIAN_POINT('Ctrl Pts',(1.03848536635828,-0.526879343018338,0.));
#4751=CARTESIAN_POINT('Ctrl Pts',(1.05296063073153,-0.499999257829972,0.));
#4752=CARTESIAN_POINT('Ctrl Pts',(1.06676816041365,-0.472733545459157,0.));
#4753=CARTESIAN_POINT('Ctrl Pts',(1.0798986829592,-0.44510073074649,0.));
#4754=CARTESIAN_POINT('Ctrl Pts',(1.09232595504273,-0.417120282666841,0.));
#4755=CARTESIAN_POINT('Ctrl Pts',(1.1040065500515,-0.388812610728411,0.));
#4756=CARTESIAN_POINT('Ctrl Pts',(1.11489509573247,-0.360198442057814,0.));
#4757=CARTESIAN_POINT('Ctrl Pts',(1.12495696400084,-0.331298301519,0.));
#4758=CARTESIAN_POINT('Ctrl Pts',(1.13418071785862,-0.302131999517994,0.));
#4759=CARTESIAN_POINT('Ctrl Pts',(1.14259364432097,-0.272718001214759,0.));
#4760=CARTESIAN_POINT('Ctrl Pts',(1.15026681194464,-0.243073201156197,0.));
#4761=CARTESIAN_POINT('Ctrl Pts',(1.15728135528338,-0.213214209193066,0.));
#4762=CARTESIAN_POINT('Ctrl Pts',(1.16370031035361,-0.183158411923726,0.));
#4763=CARTESIAN_POINT('Ctrl Pts',(1.1695394362355,-0.152925093725504,0.));
#4764=CARTESIAN_POINT('Ctrl Pts',(1.17473573615846,-0.1225365994934,0.));
#4765=CARTESIAN_POINT('Ctrl Pts',(1.17912488557723,-0.0920192855934153,
0.));
#4766=CARTESIAN_POINT('Ctrl Pts',(1.18249458653374,-0.0614026081204919,
0.));
#4767=CARTESIAN_POINT('Ctrl Pts',(1.18463081328693,-0.0307183863950716,
0.));
#4768=CARTESIAN_POINT('Ctrl Pts',(1.18536679600018,3.34053531364509E-15,
0.));
#4769=CARTESIAN_POINT('Ctrl Pts',(1.18463081328694,0.0307183863950759,0.));
#4770=CARTESIAN_POINT('Ctrl Pts',(1.18249458653375,0.0614026081204918,0.));
#4771=CARTESIAN_POINT('Ctrl Pts',(1.17912488557725,0.0920192855934129,0.));
#4772=CARTESIAN_POINT('Ctrl Pts',(1.17473573615847,0.122536599493401,0.));
#4773=CARTESIAN_POINT('Ctrl Pts',(1.1695394362355,0.152925093725509,0.));
#4774=CARTESIAN_POINT('Ctrl Pts',(1.1637003103536,0.183158411923732,0.));
#4775=CARTESIAN_POINT('Ctrl Pts',(1.15728135528336,0.21321420919307,0.));
#4776=CARTESIAN_POINT('Ctrl Pts',(1.15026681194462,0.243073201156195,0.));
#4777=CARTESIAN_POINT('Ctrl Pts',(1.14259364432096,0.272718001214758,0.));
#4778=CARTESIAN_POINT('Ctrl Pts',(1.13418071785862,0.302131999517997,0.));
#4779=CARTESIAN_POINT('Ctrl Pts',(1.12495696400085,0.33129830151901,0.));
#4780=CARTESIAN_POINT('Ctrl Pts',(1.11489509573248,0.36019844205783,0.));
#4781=CARTESIAN_POINT('Ctrl Pts',(1.10400655005151,0.388812610728428,0.));
#4782=CARTESIAN_POINT('Ctrl Pts',(1.09232595504274,0.417120282666858,0.));
#4783=CARTESIAN_POINT('Ctrl Pts',(1.0798986829592,0.4451007307465,0.));
#4784=CARTESIAN_POINT('Ctrl Pts',(1.06676816041364,0.472733545459153,0.));
#4785=CARTESIAN_POINT('Ctrl Pts',(1.05296063073151,0.499999257829953,0.));
#4786=CARTESIAN_POINT('Ctrl Pts',(1.03848536635825,0.526879343018311,0.));
#4787=CARTESIAN_POINT('Ctrl Pts',(1.02334191285218,0.553355942423933,0.));
#4788=CARTESIAN_POINT('Ctrl Pts',(1.00752529081784,0.579411667627389,0.));
#4789=CARTESIAN_POINT('Ctrl Pts',(0.991031566790874,0.605029389584491,0.));
#4790=CARTESIAN_POINT('Ctrl Pts',(0.973864462863717,0.630191986422942,0.));
#4791=CARTESIAN_POINT('Ctrl Pts',(0.956036026761713,0.654882328595531,0.));
#4792=CARTESIAN_POINT('Ctrl Pts',(0.93756331958253,0.67908342318198,0.));
#4793=CARTESIAN_POINT('Ctrl Pts',(0.918466214618686,0.702778513947035,0.));
#4794=CARTESIAN_POINT('Ctrl Pts',(0.898764943113273,0.725951191437361,0.));
#4795=CARTESIAN_POINT('Ctrl Pts',(0.87847724211534,0.748585519440939,0.));
#4796=CARTESIAN_POINT('Ctrl Pts',(0.857617760934708,0.770666069833888,0.));
#4797=CARTESIAN_POINT('Ctrl Pts',(0.836199528793927,0.792177873864058,0.));
#4798=CARTESIAN_POINT('Ctrl Pts',(0.814234876393157,0.813106395755015,0.));
#4799=CARTESIAN_POINT('Ctrl Pts',(0.79173649620936,0.833437500599952,0.));
#4800=CARTESIAN_POINT('Ctrl Pts',(0.768718652031217,0.853157416735736,0.));
#4801=CARTESIAN_POINT('Ctrl Pts',(0.745197525414833,0.872252731655753,0.));
#4802=CARTESIAN_POINT('Ctrl Pts',(0.721190552023354,0.890710427237242,0.));
#4803=CARTESIAN_POINT('Ctrl Pts',(0.696716011515856,0.908517905290589,0.));
#4804=CARTESIAN_POINT('Ctrl Pts',(0.671792549055205,0.9256630157025,0.));
#4805=CARTESIAN_POINT('Ctrl Pts',(0.64643864161945,0.942134087248967,0.));
#4806=CARTESIAN_POINT('Ctrl Pts',(0.620672396673277,0.95791994416371,0.));
#4807=CARTESIAN_POINT('Ctrl Pts',(0.594511824092183,0.973009902467561,0.));
#4808=CARTESIAN_POINT('Ctrl Pts',(0.567974995595098,0.987393771329304,0.));
#4809=CARTESIAN_POINT('Ctrl Pts',(0.541080235433915,1.00106185298108,0.));
#4810=CARTESIAN_POINT('Ctrl Pts',(0.513846332693379,1.01400494236354,0.));
#4811=CARTESIAN_POINT('Ctrl Pts',(0.486292621102429,1.02621433076829,0.));
#4812=CARTESIAN_POINT('Ctrl Pts',(0.458438841258773,1.03768181616586,0.));
#4813=CARTESIAN_POINT('Ctrl Pts',(0.430305052465076,1.04839971220046,0.));
#4814=CARTESIAN_POINT('Ctrl Pts',(0.401911530590058,1.05836085760139,0.));
#4815=CARTESIAN_POINT('Ctrl Pts',(0.373278657560858,1.06755862629372,0.));
#4816=CARTESIAN_POINT('Ctrl Pts',(0.344426864523825,1.07598693493533,0.));
#4817=CARTESIAN_POINT('Ctrl Pts',(0.315376671295687,1.08364024578392,0.));
#4818=CARTESIAN_POINT('Ctrl Pts',(0.286148704656,1.09051357088032,0.));
#4819=CARTESIAN_POINT('Ctrl Pts',(0.256763722532462,1.09660247571268,0.));
#4820=CARTESIAN_POINT('Ctrl Pts',(0.22724264215036,1.10190308368774,0.));
#4821=CARTESIAN_POINT('Ctrl Pts',(0.197606544321966,1.10641207905811,0.));
#4822=CARTESIAN_POINT('Ctrl Pts',(0.167876633777302,1.11012670736122,0.));
#4823=CARTESIAN_POINT('Ctrl Pts',(0.138074209040338,1.11304477648939,0.));
#4824=CARTESIAN_POINT('Ctrl Pts',(0.108220629786082,1.11516465787406,0.));
#4825=CARTESIAN_POINT('Ctrl Pts',(0.0783372821756164,1.11648528736656,0.));
#4826=CARTESIAN_POINT('Ctrl Pts',(0.0484455558693182,1.11700616793208,0.));
#4827=CARTESIAN_POINT('Ctrl Pts',(0.0185668417359279,1.1167273750012,0.));
#4828=CARTESIAN_POINT('Ctrl Pts',(-0.011277474795416,1.11564956182599,0.));
#4829=CARTESIAN_POINT('Ctrl Pts',(-0.041066019590905,1.11377396404697,0.));
#4830=CARTESIAN_POINT('Ctrl Pts',(-0.0707774336926752,1.11110240713063,
0.));
#4831=CARTESIAN_POINT('Ctrl Pts',(-0.100390386189687,1.10763730457062,0.));
#4832=CARTESIAN_POINT('Ctrl Pts',(-0.129883601129753,1.10338164243566,0.));
#4833=CARTESIAN_POINT('Ctrl Pts',(-0.159235881741536,1.09833896639078,0.));
#4834=CARTESIAN_POINT('Ctrl Pts',(-0.188426134393585,1.09251336987768,0.));
#4835=CARTESIAN_POINT('Ctrl Pts',(-0.217433396017983,1.08590947721851,0.));
#4836=CARTESIAN_POINT('Ctrl Pts',(-0.246236848114778,1.07853244619972,0.));
#4837=CARTESIAN_POINT('Ctrl Pts',(-0.274815813222603,1.07038799540312,0.));
#4838=CARTESIAN_POINT('Ctrl Pts',(-0.303149754470475,1.06148242804708,0.));
#4839=CARTESIAN_POINT('Ctrl Pts',(-0.3312182767774,1.05182265203972,0.));
#4840=CARTESIAN_POINT('Ctrl Pts',(-0.359001120477101,1.04141621492845,0.));
#4841=CARTESIAN_POINT('Ctrl Pts',(-0.386478184359588,1.03027128325725,0.));
#4842=CARTESIAN_POINT('Ctrl Pts',(-0.413629579915113,1.01839656305955,0.));
#4843=CARTESIAN_POINT('Ctrl Pts',(-0.440435680606144,1.00580123015714,0.));
#4844=CARTESIAN_POINT('Ctrl Pts',(-0.466877166338154,0.992494869297873,
0.));
#4845=CARTESIAN_POINT('Ctrl Pts',(-0.492935086995497,0.97848737862061,0.));
#4846=CARTESIAN_POINT('Ctrl Pts',(-0.518590849350232,0.963789014835687,
0.));
#4847=CARTESIAN_POINT('Ctrl Pts',(-0.5438261402299,0.948410555212641,0.));
#4848=CARTESIAN_POINT('Ctrl Pts',(-0.568622860345892,0.932363440835325,
0.));
#4849=CARTESIAN_POINT('Ctrl Pts',(-0.592963069825743,0.91565989731825,0.));
#4850=CARTESIAN_POINT('Ctrl Pts',(-0.616828889168791,0.898313140761531,
0.));
#4851=CARTESIAN_POINT('Ctrl Pts',(-0.64020259788639,0.880337207900991,0.));
#4852=CARTESIAN_POINT('Ctrl Pts',(-0.663066855029865,0.861746554484547,
0.));
#4853=CARTESIAN_POINT('Ctrl Pts',(-0.685404899341948,0.842555693142475,
0.));
#4854=CARTESIAN_POINT('Ctrl Pts',(-0.707200722570447,0.822778881439102,
0.));
#4855=CARTESIAN_POINT('Ctrl Pts',(-0.728439343632102,0.802429621210551,
0.));
#4856=CARTESIAN_POINT('Ctrl Pts',(-0.749106566400217,0.781521126617609,
0.));
#4857=CARTESIAN_POINT('Ctrl Pts',(-0.76918851698896,0.760067206050081,0.));
#4858=CARTESIAN_POINT('Ctrl Pts',(-0.788671222413612,0.738083066750512,
0.));
#4859=CARTESIAN_POINT('Ctrl Pts',(-0.807540237001567,0.715586030006559,
0.));
#4860=CARTESIAN_POINT('Ctrl Pts',(-0.825780081176955,0.692596598957924,
0.));
#4861=CARTESIAN_POINT('Ctrl Pts',(-0.841545334406124,0.671576597783911,
0.));
#4862=CARTESIAN_POINT('Ctrl Pts',(-0.85339188386416,0.654977418032737,0.));
#4863=CARTESIAN_POINT('Ctrl Pts',(-0.861627881959507,0.643015580660492,
0.));
#4864=CARTESIAN_POINT('Ctrl Pts',(-0.866468860926645,0.635830722731627,
0.));
#4865=CARTESIAN_POINT('Ctrl Pts',(-0.868031252847412,0.633495422775111,
0.));
#4866=CARTESIAN_POINT('',(-1.04732756983434,0.493147518935016,0.));
#4867=CARTESIAN_POINT('Origin',(-0.947327569834341,0.493147518935016,0.));
#4868=CARTESIAN_POINT('',(-1.04732756983434,-0.493147518935016,0.));
#4869=CARTESIAN_POINT('Origin',(-0.947327569834341,-0.493147518935016,0.));
#4870=CARTESIAN_POINT('Origin',(-0.947327569834341,-0.493147518935016,0.));
#4871=CARTESIAN_POINT('',(-1.04732756983434,-0.493147518935016,0.12));
#4872=CARTESIAN_POINT('',(-1.04732756983434,-0.493147518935016,0.));
#4873=CARTESIAN_POINT('Origin',(-0.947327569834341,-0.493147518935016,0.12));
#4874=CARTESIAN_POINT('Origin',(-0.947327569834341,0.493147518935016,0.));
#4875=CARTESIAN_POINT('',(-1.04732756983434,0.493147518935016,0.12));
#4876=CARTESIAN_POINT('',(-1.04732756983434,0.493147518935016,0.));
#4877=CARTESIAN_POINT('Origin',(-0.947327569834341,0.493147518935016,0.12));
#4878=CARTESIAN_POINT('Origin',(-0.947327569834341,0.493147518935016,0.));
#4879=CARTESIAN_POINT('',(-0.868031252847412,0.633495422775111,0.12));
#4880=CARTESIAN_POINT('Origin',(-0.947327569834341,0.493147518935016,0.12));
#4881=CARTESIAN_POINT('Ctrl Pts',(-0.868031252847412,0.633495422775111,
0.));
#4882=CARTESIAN_POINT('Ctrl Pts',(-0.868031252847412,0.633495422775111,
0.02));
#4883=CARTESIAN_POINT('Ctrl Pts',(-0.868031252847412,0.633495422775111,
0.04));
#4884=CARTESIAN_POINT('Ctrl Pts',(-0.868031252847412,0.633495422775111,
0.08));
#4885=CARTESIAN_POINT('Ctrl Pts',(-0.868031252847412,0.633495422775111,
0.1));
#4886=CARTESIAN_POINT('Ctrl Pts',(-0.868031252847412,0.633495422775111,
0.12));
#4887=CARTESIAN_POINT('Ctrl Pts',(-0.947327569834341,-0.493147518935016,
0.));
#4888=CARTESIAN_POINT('Ctrl Pts',(-0.947327569834341,-0.493147518935016,
0.12));
#4889=CARTESIAN_POINT('Ctrl Pts',(-0.944839172148911,-0.49844797467551,
0.));
#4890=CARTESIAN_POINT('Ctrl Pts',(-0.944839172148911,-0.49844797467551,
0.12));
#4891=CARTESIAN_POINT('Ctrl Pts',(-0.939792491218341,-0.509010207622537,
0.));
#4892=CARTESIAN_POINT('Ctrl Pts',(-0.939792491218341,-0.509010207622537,
0.12));
#4893=CARTESIAN_POINT('Ctrl Pts',(-0.932012813069913,-0.524737521565753,
0.));
#4894=CARTESIAN_POINT('Ctrl Pts',(-0.932012813069913,-0.524737521565753,
0.12));
#4895=CARTESIAN_POINT('Ctrl Pts',(-0.921220578940944,-0.545475192012581,
0.));
#4896=CARTESIAN_POINT('Ctrl Pts',(-0.921220578940944,-0.545475192012581,
0.12));
#4897=CARTESIAN_POINT('Ctrl Pts',(-0.907032039302732,-0.571009280628982,
0.));
#4898=CARTESIAN_POINT('Ctrl Pts',(-0.907032039302732,-0.571009280628982,
0.12));
#4899=CARTESIAN_POINT('Ctrl Pts',(-0.892147344045788,-0.596151853069145,
0.));
#4900=CARTESIAN_POINT('Ctrl Pts',(-0.892147344045788,-0.596151853069145,
0.12));
#4901=CARTESIAN_POINT('Ctrl Pts',(-0.876570783334336,-0.620895981731386,
0.));
#4902=CARTESIAN_POINT('Ctrl Pts',(-0.876570783334336,-0.620895981731386,
0.12));
#4903=CARTESIAN_POINT('Ctrl Pts',(-0.860309667737524,-0.645230105165021,
0.));
#4904=CARTESIAN_POINT('Ctrl Pts',(-0.860309667737524,-0.645230105165021,
0.12));
#4905=CARTESIAN_POINT('Ctrl Pts',(-0.843374934437972,-0.669137170123564,
0.));
#4906=CARTESIAN_POINT('Ctrl Pts',(-0.843374934437972,-0.669137170123564,
0.12));
#4907=CARTESIAN_POINT('Ctrl Pts',(-0.82578008117756,-0.69259659895799,0.));
#4908=CARTESIAN_POINT('Ctrl Pts',(-0.82578008117756,-0.69259659895799,0.12));
#4909=CARTESIAN_POINT('Ctrl Pts',(-0.807540237001814,-0.715586030006588,
0.));
#4910=CARTESIAN_POINT('Ctrl Pts',(-0.807540237001814,-0.715586030006588,
0.12));
#4911=CARTESIAN_POINT('Ctrl Pts',(-0.788671222413511,-0.738083066750504,
0.));
#4912=CARTESIAN_POINT('Ctrl Pts',(-0.788671222413511,-0.738083066750504,
0.12));
#4913=CARTESIAN_POINT('Ctrl Pts',(-0.769188516988648,-0.760067206050057,
0.));
#4914=CARTESIAN_POINT('Ctrl Pts',(-0.769188516988648,-0.760067206050057,
0.12));
#4915=CARTESIAN_POINT('Ctrl Pts',(-0.749106566399864,-0.781521126617586,
0.));
#4916=CARTESIAN_POINT('Ctrl Pts',(-0.749106566399864,-0.781521126617586,
0.12));
#4917=CARTESIAN_POINT('Ctrl Pts',(-0.728439343631846,-0.802429621210541,
0.));
#4918=CARTESIAN_POINT('Ctrl Pts',(-0.728439343631846,-0.802429621210541,
0.12));
#4919=CARTESIAN_POINT('Ctrl Pts',(-0.707200722570354,-0.822778881439107,
0.));
#4920=CARTESIAN_POINT('Ctrl Pts',(-0.707200722570354,-0.822778881439107,
0.12));
#4921=CARTESIAN_POINT('Ctrl Pts',(-0.685404899341998,-0.84255569314248,
0.));
#4922=CARTESIAN_POINT('Ctrl Pts',(-0.685404899341998,-0.84255569314248,
0.12));
#4923=CARTESIAN_POINT('Ctrl Pts',(-0.663066855029994,-0.861746554484541,
0.));
#4924=CARTESIAN_POINT('Ctrl Pts',(-0.663066855029994,-0.861746554484541,
0.12));
#4925=CARTESIAN_POINT('Ctrl Pts',(-0.640202597886525,-0.880337207900968,
0.));
#4926=CARTESIAN_POINT('Ctrl Pts',(-0.640202597886525,-0.880337207900968,
0.12));
#4927=CARTESIAN_POINT('Ctrl Pts',(-0.61682888916888,-0.898313140761512,
0.));
#4928=CARTESIAN_POINT('Ctrl Pts',(-0.61682888916888,-0.898313140761512,
0.12));
#4929=CARTESIAN_POINT('Ctrl Pts',(-0.592963069825771,-0.915659897318245,
0.));
#4930=CARTESIAN_POINT('Ctrl Pts',(-0.592963069825771,-0.915659897318245,
0.12));
#4931=CARTESIAN_POINT('Ctrl Pts',(-0.568622860345861,-0.932363440835334,
0.));
#4932=CARTESIAN_POINT('Ctrl Pts',(-0.568622860345861,-0.932363440835334,
0.12));
#4933=CARTESIAN_POINT('Ctrl Pts',(-0.543826140229843,-0.948410555212658,
0.));
#4934=CARTESIAN_POINT('Ctrl Pts',(-0.543826140229843,-0.948410555212658,
0.12));
#4935=CARTESIAN_POINT('Ctrl Pts',(-0.518590849350175,-0.963789014835703,
0.));
#4936=CARTESIAN_POINT('Ctrl Pts',(-0.518590849350175,-0.963789014835703,
0.12));
#4937=CARTESIAN_POINT('Ctrl Pts',(-0.492935086995462,-0.978487378620622,
0.));
#4938=CARTESIAN_POINT('Ctrl Pts',(-0.492935086995462,-0.978487378620622,
0.12));
#4939=CARTESIAN_POINT('Ctrl Pts',(-0.466877166338143,-0.992494869297879,
0.));
#4940=CARTESIAN_POINT('Ctrl Pts',(-0.466877166338143,-0.992494869297879,
0.12));
#4941=CARTESIAN_POINT('Ctrl Pts',(-0.440435680606148,-1.00580123015714,
0.));
#4942=CARTESIAN_POINT('Ctrl Pts',(-0.440435680606148,-1.00580123015714,
0.12));
#4943=CARTESIAN_POINT('Ctrl Pts',(-0.413629579915119,-1.01839656305955,
0.));
#4944=CARTESIAN_POINT('Ctrl Pts',(-0.413629579915119,-1.01839656305955,
0.12));
#4945=CARTESIAN_POINT('Ctrl Pts',(-0.386478184359591,-1.03027128325725,
0.));
#4946=CARTESIAN_POINT('Ctrl Pts',(-0.386478184359591,-1.03027128325725,
0.12));
#4947=CARTESIAN_POINT('Ctrl Pts',(-0.359001120477101,-1.04141621492846,
0.));
#4948=CARTESIAN_POINT('Ctrl Pts',(-0.359001120477101,-1.04141621492846,
0.12));
#4949=CARTESIAN_POINT('Ctrl Pts',(-0.331218276777395,-1.05182265203972,
0.));
#4950=CARTESIAN_POINT('Ctrl Pts',(-0.331218276777395,-1.05182265203972,
0.12));
#4951=CARTESIAN_POINT('Ctrl Pts',(-0.30314975447047,-1.06148242804708,0.));
#4952=CARTESIAN_POINT('Ctrl Pts',(-0.30314975447047,-1.06148242804708,0.12));
#4953=CARTESIAN_POINT('Ctrl Pts',(-0.2748158132226,-1.07038799540312,0.));
#4954=CARTESIAN_POINT('Ctrl Pts',(-0.2748158132226,-1.07038799540312,0.12));
#4955=CARTESIAN_POINT('Ctrl Pts',(-0.246236848114779,-1.07853244619974,
0.));
#4956=CARTESIAN_POINT('Ctrl Pts',(-0.246236848114779,-1.07853244619974,
0.12));
#4957=CARTESIAN_POINT('Ctrl Pts',(-0.217433396017985,-1.08590947721852,
0.));
#4958=CARTESIAN_POINT('Ctrl Pts',(-0.217433396017985,-1.08590947721852,
0.12));
#4959=CARTESIAN_POINT('Ctrl Pts',(-0.188426134393584,-1.09251336987768,
0.));
#4960=CARTESIAN_POINT('Ctrl Pts',(-0.188426134393584,-1.09251336987768,
0.12));
#4961=CARTESIAN_POINT('Ctrl Pts',(-0.159235881741527,-1.09833896639077,
0.));
#4962=CARTESIAN_POINT('Ctrl Pts',(-0.159235881741527,-1.09833896639077,
0.12));
#4963=CARTESIAN_POINT('Ctrl Pts',(-0.129883601129733,-1.10338164243564,
0.));
#4964=CARTESIAN_POINT('Ctrl Pts',(-0.129883601129733,-1.10338164243564,
0.12));
#4965=CARTESIAN_POINT('Ctrl Pts',(-0.100390386189668,-1.1076373045706,0.));
#4966=CARTESIAN_POINT('Ctrl Pts',(-0.100390386189668,-1.1076373045706,0.12));
#4967=CARTESIAN_POINT('Ctrl Pts',(-0.0707774336926613,-1.11110240713062,
0.));
#4968=CARTESIAN_POINT('Ctrl Pts',(-0.0707774336926613,-1.11110240713062,
0.12));
#4969=CARTESIAN_POINT('Ctrl Pts',(-0.0410660195909007,-1.11377396404697,
0.));
#4970=CARTESIAN_POINT('Ctrl Pts',(-0.0410660195909007,-1.11377396404697,
0.12));
#4971=CARTESIAN_POINT('Ctrl Pts',(-0.0112774747954127,-1.11564956182599,
0.));
#4972=CARTESIAN_POINT('Ctrl Pts',(-0.0112774747954127,-1.11564956182599,
0.12));
#4973=CARTESIAN_POINT('Ctrl Pts',(0.0185668417359402,-1.11672737500119,
0.));
#4974=CARTESIAN_POINT('Ctrl Pts',(0.0185668417359402,-1.11672737500119,
0.12));
#4975=CARTESIAN_POINT('Ctrl Pts',(0.0484455558693415,-1.11700616793207,
0.));
#4976=CARTESIAN_POINT('Ctrl Pts',(0.0484455558693415,-1.11700616793207,
0.12));
#4977=CARTESIAN_POINT('Ctrl Pts',(0.0783372821756426,-1.11648528736655,
0.));
#4978=CARTESIAN_POINT('Ctrl Pts',(0.0783372821756426,-1.11648528736655,
0.12));
#4979=CARTESIAN_POINT('Ctrl Pts',(0.108220629786098,-1.11516465787405,0.));
#4980=CARTESIAN_POINT('Ctrl Pts',(0.108220629786098,-1.11516465787405,0.12));
#4981=CARTESIAN_POINT('Ctrl Pts',(0.138074209040328,-1.1130447764894,0.));
#4982=CARTESIAN_POINT('Ctrl Pts',(0.138074209040328,-1.1130447764894,0.12));
#4983=CARTESIAN_POINT('Ctrl Pts',(0.167876633777266,-1.11012670736124,0.));
#4984=CARTESIAN_POINT('Ctrl Pts',(0.167876633777266,-1.11012670736124,0.12));
#4985=CARTESIAN_POINT('Ctrl Pts',(0.197606544321918,-1.10641207905813,0.));
#4986=CARTESIAN_POINT('Ctrl Pts',(0.197606544321918,-1.10641207905813,0.12));
#4987=CARTESIAN_POINT('Ctrl Pts',(0.227242642150327,-1.10190308368776,0.));
#4988=CARTESIAN_POINT('Ctrl Pts',(0.227242642150327,-1.10190308368776,0.12));
#4989=CARTESIAN_POINT('Ctrl Pts',(0.256763722532457,-1.09660247571268,0.));
#4990=CARTESIAN_POINT('Ctrl Pts',(0.256763722532457,-1.09660247571268,0.12));
#4991=CARTESIAN_POINT('Ctrl Pts',(0.286148704656023,-1.09051357088032,0.));
#4992=CARTESIAN_POINT('Ctrl Pts',(0.286148704656023,-1.09051357088032,0.12));
#4993=CARTESIAN_POINT('Ctrl Pts',(0.315376671295726,-1.08364024578391,0.));
#4994=CARTESIAN_POINT('Ctrl Pts',(0.315376671295726,-1.08364024578391,0.12));
#4995=CARTESIAN_POINT('Ctrl Pts',(0.344426864523868,-1.07598693493533,0.));
#4996=CARTESIAN_POINT('Ctrl Pts',(0.344426864523868,-1.07598693493533,0.12));
#4997=CARTESIAN_POINT('Ctrl Pts',(0.373278657560889,-1.06755862629372,0.));
#4998=CARTESIAN_POINT('Ctrl Pts',(0.373278657560889,-1.06755862629372,0.12));
#4999=CARTESIAN_POINT('Ctrl Pts',(0.40191153059007,-1.05836085760139,0.));
#5000=CARTESIAN_POINT('Ctrl Pts',(0.40191153059007,-1.05836085760139,0.12));
#5001=CARTESIAN_POINT('Ctrl Pts',(0.430305052465067,-1.04839971220046,0.));
#5002=CARTESIAN_POINT('Ctrl Pts',(0.430305052465067,-1.04839971220046,0.12));
#5003=CARTESIAN_POINT('Ctrl Pts',(0.45843884125875,-1.03768181616585,0.));
#5004=CARTESIAN_POINT('Ctrl Pts',(0.45843884125875,-1.03768181616585,0.12));
#5005=CARTESIAN_POINT('Ctrl Pts',(0.486292621102405,-1.02621433076827,0.));
#5006=CARTESIAN_POINT('Ctrl Pts',(0.486292621102405,-1.02621433076827,0.12));
#5007=CARTESIAN_POINT('Ctrl Pts',(0.513846332693361,-1.01400494236352,0.));
#5008=CARTESIAN_POINT('Ctrl Pts',(0.513846332693361,-1.01400494236352,0.12));
#5009=CARTESIAN_POINT('Ctrl Pts',(0.541080235433912,-1.00106185298107,0.));
#5010=CARTESIAN_POINT('Ctrl Pts',(0.541080235433912,-1.00106185298107,0.12));
#5011=CARTESIAN_POINT('Ctrl Pts',(0.567974995595113,-0.987393771329312,
0.));
#5012=CARTESIAN_POINT('Ctrl Pts',(0.567974995595113,-0.987393771329312,
0.12));
#5013=CARTESIAN_POINT('Ctrl Pts',(0.594511824092215,-0.973009902467593,
0.));
#5014=CARTESIAN_POINT('Ctrl Pts',(0.594511824092215,-0.973009902467593,
0.12));
#5015=CARTESIAN_POINT('Ctrl Pts',(0.620672396673315,-0.957919944163756,
0.));
#5016=CARTESIAN_POINT('Ctrl Pts',(0.620672396673315,-0.957919944163756,
0.12));
#5017=CARTESIAN_POINT('Ctrl Pts',(0.646438641619482,-0.942134087249009,
0.));
#5018=CARTESIAN_POINT('Ctrl Pts',(0.646438641619482,-0.942134087249009,
0.12));
#5019=CARTESIAN_POINT('Ctrl Pts',(0.67179254905522,-0.925663015702513,0.));
#5020=CARTESIAN_POINT('Ctrl Pts',(0.67179254905522,-0.925663015702513,0.12));
#5021=CARTESIAN_POINT('Ctrl Pts',(0.696716011515847,-0.908517905290565,
0.));
#5022=CARTESIAN_POINT('Ctrl Pts',(0.696716011515847,-0.908517905290565,
0.12));
#5023=CARTESIAN_POINT('Ctrl Pts',(0.721190552023322,-0.890710427237186,
0.));
#5024=CARTESIAN_POINT('Ctrl Pts',(0.721190552023322,-0.890710427237186,
0.12));
#5025=CARTESIAN_POINT('Ctrl Pts',(0.745197525414791,-0.872252731655685,
0.));
#5026=CARTESIAN_POINT('Ctrl Pts',(0.745197525414791,-0.872252731655685,
0.12));
#5027=CARTESIAN_POINT('Ctrl Pts',(0.768718652031186,-0.853157416735685,
0.));
#5028=CARTESIAN_POINT('Ctrl Pts',(0.768718652031186,-0.853157416735685,
0.12));
#5029=CARTESIAN_POINT('Ctrl Pts',(0.791736496209353,-0.833437500599933,
0.));
#5030=CARTESIAN_POINT('Ctrl Pts',(0.791736496209353,-0.833437500599933,
0.12));
#5031=CARTESIAN_POINT('Ctrl Pts',(0.814234876393174,-0.81310639575503,0.));
#5032=CARTESIAN_POINT('Ctrl Pts',(0.814234876393174,-0.81310639575503,0.12));
#5033=CARTESIAN_POINT('Ctrl Pts',(0.836199528793963,-0.792177873864096,
0.));
#5034=CARTESIAN_POINT('Ctrl Pts',(0.836199528793963,-0.792177873864096,
0.12));
#5035=CARTESIAN_POINT('Ctrl Pts',(0.857617760934752,-0.770666069833932,
0.));
#5036=CARTESIAN_POINT('Ctrl Pts',(0.857617760934752,-0.770666069833932,
0.12));
#5037=CARTESIAN_POINT('Ctrl Pts',(0.878477242115376,-0.74858551944097,0.));
#5038=CARTESIAN_POINT('Ctrl Pts',(0.878477242115376,-0.74858551944097,0.12));
#5039=CARTESIAN_POINT('Ctrl Pts',(0.898764943113291,-0.725951191437368,
0.));
#5040=CARTESIAN_POINT('Ctrl Pts',(0.898764943113291,-0.725951191437368,
0.12));
#5041=CARTESIAN_POINT('Ctrl Pts',(0.918466214618678,-0.70277851394702,0.));
#5042=CARTESIAN_POINT('Ctrl Pts',(0.918466214618678,-0.70277851394702,0.12));
#5043=CARTESIAN_POINT('Ctrl Pts',(0.937563319582499,-0.679083423181946,
0.));
#5044=CARTESIAN_POINT('Ctrl Pts',(0.937563319582499,-0.679083423181946,
0.12));
#5045=CARTESIAN_POINT('Ctrl Pts',(0.956036026761672,-0.654882328595489,
0.));
#5046=CARTESIAN_POINT('Ctrl Pts',(0.956036026761672,-0.654882328595489,
0.12));
#5047=CARTESIAN_POINT('Ctrl Pts',(0.973864462863685,-0.630191986422907,
0.));
#5048=CARTESIAN_POINT('Ctrl Pts',(0.973864462863685,-0.630191986422907,
0.12));
#5049=CARTESIAN_POINT('Ctrl Pts',(0.991031566790864,-0.605029389584474,
0.));
#5050=CARTESIAN_POINT('Ctrl Pts',(0.991031566790864,-0.605029389584474,
0.12));
#5051=CARTESIAN_POINT('Ctrl Pts',(1.00752529081786,-0.579411667627393,0.));
#5052=CARTESIAN_POINT('Ctrl Pts',(1.00752529081786,-0.579411667627393,0.12));
#5053=CARTESIAN_POINT('Ctrl Pts',(1.02334191285221,-0.553355942423953,0.));
#5054=CARTESIAN_POINT('Ctrl Pts',(1.02334191285221,-0.553355942423953,0.12));
#5055=CARTESIAN_POINT('Ctrl Pts',(1.03848536635828,-0.526879343018338,0.));
#5056=CARTESIAN_POINT('Ctrl Pts',(1.03848536635828,-0.526879343018338,0.12));
#5057=CARTESIAN_POINT('Ctrl Pts',(1.05296063073153,-0.499999257829972,0.));
#5058=CARTESIAN_POINT('Ctrl Pts',(1.05296063073153,-0.499999257829972,0.12));
#5059=CARTESIAN_POINT('Ctrl Pts',(1.06676816041365,-0.472733545459157,0.));
#5060=CARTESIAN_POINT('Ctrl Pts',(1.06676816041365,-0.472733545459157,0.12));
#5061=CARTESIAN_POINT('Ctrl Pts',(1.0798986829592,-0.44510073074649,0.));
#5062=CARTESIAN_POINT('Ctrl Pts',(1.0798986829592,-0.44510073074649,0.12));
#5063=CARTESIAN_POINT('Ctrl Pts',(1.09232595504273,-0.417120282666841,0.));
#5064=CARTESIAN_POINT('Ctrl Pts',(1.09232595504273,-0.417120282666841,0.12));
#5065=CARTESIAN_POINT('Ctrl Pts',(1.1040065500515,-0.388812610728411,0.));
#5066=CARTESIAN_POINT('Ctrl Pts',(1.1040065500515,-0.388812610728411,0.12));
#5067=CARTESIAN_POINT('Ctrl Pts',(1.11489509573247,-0.360198442057814,0.));
#5068=CARTESIAN_POINT('Ctrl Pts',(1.11489509573247,-0.360198442057814,0.12));
#5069=CARTESIAN_POINT('Ctrl Pts',(1.12495696400084,-0.331298301519,0.));
#5070=CARTESIAN_POINT('Ctrl Pts',(1.12495696400084,-0.331298301519,0.12));
#5071=CARTESIAN_POINT('Ctrl Pts',(1.13418071785862,-0.302131999517994,0.));
#5072=CARTESIAN_POINT('Ctrl Pts',(1.13418071785862,-0.302131999517994,0.12));
#5073=CARTESIAN_POINT('Ctrl Pts',(1.14259364432097,-0.272718001214759,0.));
#5074=CARTESIAN_POINT('Ctrl Pts',(1.14259364432097,-0.272718001214759,0.12));
#5075=CARTESIAN_POINT('Ctrl Pts',(1.15026681194464,-0.243073201156197,0.));
#5076=CARTESIAN_POINT('Ctrl Pts',(1.15026681194464,-0.243073201156197,0.12));
#5077=CARTESIAN_POINT('Ctrl Pts',(1.15728135528338,-0.213214209193066,0.));
#5078=CARTESIAN_POINT('Ctrl Pts',(1.15728135528338,-0.213214209193066,0.12));
#5079=CARTESIAN_POINT('Ctrl Pts',(1.16370031035361,-0.183158411923726,0.));
#5080=CARTESIAN_POINT('Ctrl Pts',(1.16370031035361,-0.183158411923726,0.12));
#5081=CARTESIAN_POINT('Ctrl Pts',(1.1695394362355,-0.152925093725504,0.));
#5082=CARTESIAN_POINT('Ctrl Pts',(1.1695394362355,-0.152925093725504,0.12));
#5083=CARTESIAN_POINT('Ctrl Pts',(1.17473573615846,-0.1225365994934,0.));
#5084=CARTESIAN_POINT('Ctrl Pts',(1.17473573615846,-0.1225365994934,0.12));
#5085=CARTESIAN_POINT('Ctrl Pts',(1.17912488557723,-0.0920192855934153,
0.));
#5086=CARTESIAN_POINT('Ctrl Pts',(1.17912488557723,-0.0920192855934153,
0.12));
#5087=CARTESIAN_POINT('Ctrl Pts',(1.18249458653374,-0.0614026081204919,
0.));
#5088=CARTESIAN_POINT('Ctrl Pts',(1.18249458653374,-0.0614026081204919,
0.12));
#5089=CARTESIAN_POINT('Ctrl Pts',(1.18463081328693,-0.0307183863950716,
0.));
#5090=CARTESIAN_POINT('Ctrl Pts',(1.18463081328693,-0.0307183863950716,
0.12));
#5091=CARTESIAN_POINT('Ctrl Pts',(1.18536679600018,3.34053531364509E-15,
0.));
#5092=CARTESIAN_POINT('Ctrl Pts',(1.18536679600018,3.34053531364509E-15,
0.12));
#5093=CARTESIAN_POINT('Ctrl Pts',(1.18463081328694,0.0307183863950759,0.));
#5094=CARTESIAN_POINT('Ctrl Pts',(1.18463081328694,0.0307183863950759,0.12));
#5095=CARTESIAN_POINT('Ctrl Pts',(1.18249458653375,0.0614026081204918,0.));
#5096=CARTESIAN_POINT('Ctrl Pts',(1.18249458653375,0.0614026081204918,0.12));
#5097=CARTESIAN_POINT('Ctrl Pts',(1.17912488557725,0.0920192855934129,0.));
#5098=CARTESIAN_POINT('Ctrl Pts',(1.17912488557725,0.0920192855934129,0.12));
#5099=CARTESIAN_POINT('Ctrl Pts',(1.17473573615847,0.122536599493401,0.));
#5100=CARTESIAN_POINT('Ctrl Pts',(1.17473573615847,0.122536599493401,0.12));
#5101=CARTESIAN_POINT('Ctrl Pts',(1.1695394362355,0.152925093725509,0.));
#5102=CARTESIAN_POINT('Ctrl Pts',(1.1695394362355,0.152925093725509,0.12));
#5103=CARTESIAN_POINT('Ctrl Pts',(1.1637003103536,0.183158411923732,0.));
#5104=CARTESIAN_POINT('Ctrl Pts',(1.1637003103536,0.183158411923732,0.12));
#5105=CARTESIAN_POINT('Ctrl Pts',(1.15728135528336,0.21321420919307,0.));
#5106=CARTESIAN_POINT('Ctrl Pts',(1.15728135528336,0.21321420919307,0.12));
#5107=CARTESIAN_POINT('Ctrl Pts',(1.15026681194462,0.243073201156195,0.));
#5108=CARTESIAN_POINT('Ctrl Pts',(1.15026681194462,0.243073201156195,0.12));
#5109=CARTESIAN_POINT('Ctrl Pts',(1.14259364432096,0.272718001214758,0.));
#5110=CARTESIAN_POINT('Ctrl Pts',(1.14259364432096,0.272718001214758,0.12));
#5111=CARTESIAN_POINT('Ctrl Pts',(1.13418071785862,0.302131999517997,0.));
#5112=CARTESIAN_POINT('Ctrl Pts',(1.13418071785862,0.302131999517997,0.12));
#5113=CARTESIAN_POINT('Ctrl Pts',(1.12495696400085,0.33129830151901,0.));
#5114=CARTESIAN_POINT('Ctrl Pts',(1.12495696400085,0.33129830151901,0.12));
#5115=CARTESIAN_POINT('Ctrl Pts',(1.11489509573248,0.36019844205783,0.));
#5116=CARTESIAN_POINT('Ctrl Pts',(1.11489509573248,0.36019844205783,0.12));
#5117=CARTESIAN_POINT('Ctrl Pts',(1.10400655005151,0.388812610728428,0.));
#5118=CARTESIAN_POINT('Ctrl Pts',(1.10400655005151,0.388812610728428,0.12));
#5119=CARTESIAN_POINT('Ctrl Pts',(1.09232595504274,0.417120282666858,0.));
#5120=CARTESIAN_POINT('Ctrl Pts',(1.09232595504274,0.417120282666858,0.12));
#5121=CARTESIAN_POINT('Ctrl Pts',(1.0798986829592,0.4451007307465,0.));
#5122=CARTESIAN_POINT('Ctrl Pts',(1.0798986829592,0.4451007307465,0.12));
#5123=CARTESIAN_POINT('Ctrl Pts',(1.06676816041364,0.472733545459153,0.));
#5124=CARTESIAN_POINT('Ctrl Pts',(1.06676816041364,0.472733545459153,0.12));
#5125=CARTESIAN_POINT('Ctrl Pts',(1.05296063073151,0.499999257829953,0.));
#5126=CARTESIAN_POINT('Ctrl Pts',(1.05296063073151,0.499999257829953,0.12));
#5127=CARTESIAN_POINT('Ctrl Pts',(1.03848536635825,0.526879343018311,0.));
#5128=CARTESIAN_POINT('Ctrl Pts',(1.03848536635825,0.526879343018311,0.12));
#5129=CARTESIAN_POINT('Ctrl Pts',(1.02334191285218,0.553355942423933,0.));
#5130=CARTESIAN_POINT('Ctrl Pts',(1.02334191285218,0.553355942423933,0.12));
#5131=CARTESIAN_POINT('Ctrl Pts',(1.00752529081784,0.579411667627389,0.));
#5132=CARTESIAN_POINT('Ctrl Pts',(1.00752529081784,0.579411667627389,0.12));
#5133=CARTESIAN_POINT('Ctrl Pts',(0.991031566790874,0.605029389584491,0.));
#5134=CARTESIAN_POINT('Ctrl Pts',(0.991031566790874,0.605029389584491,0.12));
#5135=CARTESIAN_POINT('Ctrl Pts',(0.973864462863717,0.630191986422942,0.));
#5136=CARTESIAN_POINT('Ctrl Pts',(0.973864462863717,0.630191986422942,0.12));
#5137=CARTESIAN_POINT('Ctrl Pts',(0.956036026761713,0.654882328595531,0.));
#5138=CARTESIAN_POINT('Ctrl Pts',(0.956036026761713,0.654882328595531,0.12));
#5139=CARTESIAN_POINT('Ctrl Pts',(0.93756331958253,0.67908342318198,0.));
#5140=CARTESIAN_POINT('Ctrl Pts',(0.93756331958253,0.67908342318198,0.12));
#5141=CARTESIAN_POINT('Ctrl Pts',(0.918466214618686,0.702778513947035,0.));
#5142=CARTESIAN_POINT('Ctrl Pts',(0.918466214618686,0.702778513947035,0.12));
#5143=CARTESIAN_POINT('Ctrl Pts',(0.898764943113273,0.725951191437361,0.));
#5144=CARTESIAN_POINT('Ctrl Pts',(0.898764943113273,0.725951191437361,0.12));
#5145=CARTESIAN_POINT('Ctrl Pts',(0.87847724211534,0.748585519440939,0.));
#5146=CARTESIAN_POINT('Ctrl Pts',(0.87847724211534,0.748585519440939,0.12));
#5147=CARTESIAN_POINT('Ctrl Pts',(0.857617760934708,0.770666069833888,0.));
#5148=CARTESIAN_POINT('Ctrl Pts',(0.857617760934708,0.770666069833888,0.12));
#5149=CARTESIAN_POINT('Ctrl Pts',(0.836199528793927,0.792177873864058,0.));
#5150=CARTESIAN_POINT('Ctrl Pts',(0.836199528793927,0.792177873864058,0.12));
#5151=CARTESIAN_POINT('Ctrl Pts',(0.814234876393157,0.813106395755015,0.));
#5152=CARTESIAN_POINT('Ctrl Pts',(0.814234876393157,0.813106395755015,0.12));
#5153=CARTESIAN_POINT('Ctrl Pts',(0.79173649620936,0.833437500599952,0.));
#5154=CARTESIAN_POINT('Ctrl Pts',(0.79173649620936,0.833437500599952,0.12));
#5155=CARTESIAN_POINT('Ctrl Pts',(0.768718652031217,0.853157416735736,0.));
#5156=CARTESIAN_POINT('Ctrl Pts',(0.768718652031217,0.853157416735736,0.12));
#5157=CARTESIAN_POINT('Ctrl Pts',(0.745197525414833,0.872252731655753,0.));
#5158=CARTESIAN_POINT('Ctrl Pts',(0.745197525414833,0.872252731655753,0.12));
#5159=CARTESIAN_POINT('Ctrl Pts',(0.721190552023354,0.890710427237242,0.));
#5160=CARTESIAN_POINT('Ctrl Pts',(0.721190552023354,0.890710427237242,0.12));
#5161=CARTESIAN_POINT('Ctrl Pts',(0.696716011515856,0.908517905290589,0.));
#5162=CARTESIAN_POINT('Ctrl Pts',(0.696716011515856,0.908517905290589,0.12));
#5163=CARTESIAN_POINT('Ctrl Pts',(0.671792549055205,0.9256630157025,0.));
#5164=CARTESIAN_POINT('Ctrl Pts',(0.671792549055205,0.9256630157025,0.12));
#5165=CARTESIAN_POINT('Ctrl Pts',(0.64643864161945,0.942134087248967,0.));
#5166=CARTESIAN_POINT('Ctrl Pts',(0.64643864161945,0.942134087248967,0.12));
#5167=CARTESIAN_POINT('Ctrl Pts',(0.620672396673277,0.95791994416371,0.));
#5168=CARTESIAN_POINT('Ctrl Pts',(0.620672396673277,0.95791994416371,0.12));
#5169=CARTESIAN_POINT('Ctrl Pts',(0.594511824092183,0.973009902467561,0.));
#5170=CARTESIAN_POINT('Ctrl Pts',(0.594511824092183,0.973009902467561,0.12));
#5171=CARTESIAN_POINT('Ctrl Pts',(0.567974995595098,0.987393771329304,0.));
#5172=CARTESIAN_POINT('Ctrl Pts',(0.567974995595098,0.987393771329304,0.12));
#5173=CARTESIAN_POINT('Ctrl Pts',(0.541080235433915,1.00106185298108,0.));
#5174=CARTESIAN_POINT('Ctrl Pts',(0.541080235433915,1.00106185298108,0.12));
#5175=CARTESIAN_POINT('Ctrl Pts',(0.513846332693379,1.01400494236354,0.));
#5176=CARTESIAN_POINT('Ctrl Pts',(0.513846332693379,1.01400494236354,0.12));
#5177=CARTESIAN_POINT('Ctrl Pts',(0.486292621102429,1.02621433076829,0.));
#5178=CARTESIAN_POINT('Ctrl Pts',(0.486292621102429,1.02621433076829,0.12));
#5179=CARTESIAN_POINT('Ctrl Pts',(0.458438841258773,1.03768181616586,0.));
#5180=CARTESIAN_POINT('Ctrl Pts',(0.458438841258773,1.03768181616586,0.12));
#5181=CARTESIAN_POINT('Ctrl Pts',(0.430305052465076,1.04839971220046,0.));
#5182=CARTESIAN_POINT('Ctrl Pts',(0.430305052465076,1.04839971220046,0.12));
#5183=CARTESIAN_POINT('Ctrl Pts',(0.401911530590058,1.05836085760139,0.));
#5184=CARTESIAN_POINT('Ctrl Pts',(0.401911530590058,1.05836085760139,0.12));
#5185=CARTESIAN_POINT('Ctrl Pts',(0.373278657560858,1.06755862629372,0.));
#5186=CARTESIAN_POINT('Ctrl Pts',(0.373278657560858,1.06755862629372,0.12));
#5187=CARTESIAN_POINT('Ctrl Pts',(0.344426864523825,1.07598693493533,0.));
#5188=CARTESIAN_POINT('Ctrl Pts',(0.344426864523825,1.07598693493533,0.12));
#5189=CARTESIAN_POINT('Ctrl Pts',(0.315376671295687,1.08364024578392,0.));
#5190=CARTESIAN_POINT('Ctrl Pts',(0.315376671295687,1.08364024578392,0.12));
#5191=CARTESIAN_POINT('Ctrl Pts',(0.286148704656,1.09051357088032,0.));
#5192=CARTESIAN_POINT('Ctrl Pts',(0.286148704656,1.09051357088032,0.12));
#5193=CARTESIAN_POINT('Ctrl Pts',(0.256763722532462,1.09660247571268,0.));
#5194=CARTESIAN_POINT('Ctrl Pts',(0.256763722532462,1.09660247571268,0.12));
#5195=CARTESIAN_POINT('Ctrl Pts',(0.22724264215036,1.10190308368774,0.));
#5196=CARTESIAN_POINT('Ctrl Pts',(0.22724264215036,1.10190308368774,0.12));
#5197=CARTESIAN_POINT('Ctrl Pts',(0.197606544321966,1.10641207905811,0.));
#5198=CARTESIAN_POINT('Ctrl Pts',(0.197606544321966,1.10641207905811,0.12));
#5199=CARTESIAN_POINT('Ctrl Pts',(0.167876633777302,1.11012670736122,0.));
#5200=CARTESIAN_POINT('Ctrl Pts',(0.167876633777302,1.11012670736122,0.12));
#5201=CARTESIAN_POINT('Ctrl Pts',(0.138074209040338,1.11304477648939,0.));
#5202=CARTESIAN_POINT('Ctrl Pts',(0.138074209040338,1.11304477648939,0.12));
#5203=CARTESIAN_POINT('Ctrl Pts',(0.108220629786082,1.11516465787406,0.));
#5204=CARTESIAN_POINT('Ctrl Pts',(0.108220629786082,1.11516465787406,0.12));
#5205=CARTESIAN_POINT('Ctrl Pts',(0.0783372821756164,1.11648528736656,0.));
#5206=CARTESIAN_POINT('Ctrl Pts',(0.0783372821756164,1.11648528736656,0.12));
#5207=CARTESIAN_POINT('Ctrl Pts',(0.0484455558693182,1.11700616793208,0.));
#5208=CARTESIAN_POINT('Ctrl Pts',(0.0484455558693182,1.11700616793208,0.12));
#5209=CARTESIAN_POINT('Ctrl Pts',(0.0185668417359279,1.1167273750012,0.));
#5210=CARTESIAN_POINT('Ctrl Pts',(0.0185668417359279,1.1167273750012,0.12));
#5211=CARTESIAN_POINT('Ctrl Pts',(-0.011277474795416,1.11564956182599,0.));
#5212=CARTESIAN_POINT('Ctrl Pts',(-0.011277474795416,1.11564956182599,0.12));
#5213=CARTESIAN_POINT('Ctrl Pts',(-0.041066019590905,1.11377396404697,0.));
#5214=CARTESIAN_POINT('Ctrl Pts',(-0.041066019590905,1.11377396404697,0.12));
#5215=CARTESIAN_POINT('Ctrl Pts',(-0.0707774336926752,1.11110240713063,
0.));
#5216=CARTESIAN_POINT('Ctrl Pts',(-0.0707774336926752,1.11110240713063,
0.12));
#5217=CARTESIAN_POINT('Ctrl Pts',(-0.100390386189687,1.10763730457062,0.));
#5218=CARTESIAN_POINT('Ctrl Pts',(-0.100390386189687,1.10763730457062,0.12));
#5219=CARTESIAN_POINT('Ctrl Pts',(-0.129883601129753,1.10338164243566,0.));
#5220=CARTESIAN_POINT('Ctrl Pts',(-0.129883601129753,1.10338164243566,0.12));
#5221=CARTESIAN_POINT('Ctrl Pts',(-0.159235881741536,1.09833896639078,0.));
#5222=CARTESIAN_POINT('Ctrl Pts',(-0.159235881741536,1.09833896639078,0.12));
#5223=CARTESIAN_POINT('Ctrl Pts',(-0.188426134393585,1.09251336987768,0.));
#5224=CARTESIAN_POINT('Ctrl Pts',(-0.188426134393585,1.09251336987768,0.12));
#5225=CARTESIAN_POINT('Ctrl Pts',(-0.217433396017983,1.08590947721851,0.));
#5226=CARTESIAN_POINT('Ctrl Pts',(-0.217433396017983,1.08590947721851,0.12));
#5227=CARTESIAN_POINT('Ctrl Pts',(-0.246236848114778,1.07853244619972,0.));
#5228=CARTESIAN_POINT('Ctrl Pts',(-0.246236848114778,1.07853244619972,0.12));
#5229=CARTESIAN_POINT('Ctrl Pts',(-0.274815813222603,1.07038799540312,0.));
#5230=CARTESIAN_POINT('Ctrl Pts',(-0.274815813222603,1.07038799540312,0.12));
#5231=CARTESIAN_POINT('Ctrl Pts',(-0.303149754470475,1.06148242804708,0.));
#5232=CARTESIAN_POINT('Ctrl Pts',(-0.303149754470475,1.06148242804708,0.12));
#5233=CARTESIAN_POINT('Ctrl Pts',(-0.3312182767774,1.05182265203972,0.));
#5234=CARTESIAN_POINT('Ctrl Pts',(-0.3312182767774,1.05182265203972,0.12));
#5235=CARTESIAN_POINT('Ctrl Pts',(-0.359001120477101,1.04141621492845,0.));
#5236=CARTESIAN_POINT('Ctrl Pts',(-0.359001120477101,1.04141621492845,0.12));
#5237=CARTESIAN_POINT('Ctrl Pts',(-0.386478184359588,1.03027128325725,0.));
#5238=CARTESIAN_POINT('Ctrl Pts',(-0.386478184359588,1.03027128325725,0.12));
#5239=CARTESIAN_POINT('Ctrl Pts',(-0.413629579915113,1.01839656305955,0.));
#5240=CARTESIAN_POINT('Ctrl Pts',(-0.413629579915113,1.01839656305955,0.12));
#5241=CARTESIAN_POINT('Ctrl Pts',(-0.440435680606144,1.00580123015714,0.));
#5242=CARTESIAN_POINT('Ctrl Pts',(-0.440435680606144,1.00580123015714,0.12));
#5243=CARTESIAN_POINT('Ctrl Pts',(-0.466877166338154,0.992494869297873,
0.));
#5244=CARTESIAN_POINT('Ctrl Pts',(-0.466877166338154,0.992494869297873,
0.12));
#5245=CARTESIAN_POINT('Ctrl Pts',(-0.492935086995497,0.97848737862061,0.));
#5246=CARTESIAN_POINT('Ctrl Pts',(-0.492935086995497,0.97848737862061,0.12));
#5247=CARTESIAN_POINT('Ctrl Pts',(-0.518590849350232,0.963789014835687,
0.));
#5248=CARTESIAN_POINT('Ctrl Pts',(-0.518590849350232,0.963789014835687,
0.12));
#5249=CARTESIAN_POINT('Ctrl Pts',(-0.5438261402299,0.948410555212641,0.));
#5250=CARTESIAN_POINT('Ctrl Pts',(-0.5438261402299,0.948410555212641,0.12));
#5251=CARTESIAN_POINT('Ctrl Pts',(-0.568622860345892,0.932363440835325,
0.));
#5252=CARTESIAN_POINT('Ctrl Pts',(-0.568622860345892,0.932363440835325,
0.12));
#5253=CARTESIAN_POINT('Ctrl Pts',(-0.592963069825743,0.91565989731825,0.));
#5254=CARTESIAN_POINT('Ctrl Pts',(-0.592963069825743,0.91565989731825,0.12));
#5255=CARTESIAN_POINT('Ctrl Pts',(-0.616828889168791,0.898313140761531,
0.));
#5256=CARTESIAN_POINT('Ctrl Pts',(-0.616828889168791,0.898313140761531,
0.12));
#5257=CARTESIAN_POINT('Ctrl Pts',(-0.64020259788639,0.880337207900991,0.));
#5258=CARTESIAN_POINT('Ctrl Pts',(-0.64020259788639,0.880337207900991,0.12));
#5259=CARTESIAN_POINT('Ctrl Pts',(-0.663066855029865,0.861746554484547,
0.));
#5260=CARTESIAN_POINT('Ctrl Pts',(-0.663066855029865,0.861746554484547,
0.12));
#5261=CARTESIAN_POINT('Ctrl Pts',(-0.685404899341948,0.842555693142475,
0.));
#5262=CARTESIAN_POINT('Ctrl Pts',(-0.685404899341948,0.842555693142475,
0.12));
#5263=CARTESIAN_POINT('Ctrl Pts',(-0.707200722570447,0.822778881439102,
0.));
#5264=CARTESIAN_POINT('Ctrl Pts',(-0.707200722570447,0.822778881439102,
0.12));
#5265=CARTESIAN_POINT('Ctrl Pts',(-0.728439343632102,0.802429621210551,
0.));
#5266=CARTESIAN_POINT('Ctrl Pts',(-0.728439343632102,0.802429621210551,
0.12));
#5267=CARTESIAN_POINT('Ctrl Pts',(-0.749106566400217,0.781521126617609,
0.));
#5268=CARTESIAN_POINT('Ctrl Pts',(-0.749106566400217,0.781521126617609,
0.12));
#5269=CARTESIAN_POINT('Ctrl Pts',(-0.76918851698896,0.760067206050081,0.));
#5270=CARTESIAN_POINT('Ctrl Pts',(-0.76918851698896,0.760067206050081,0.12));
#5271=CARTESIAN_POINT('Ctrl Pts',(-0.788671222413612,0.738083066750512,
0.));
#5272=CARTESIAN_POINT('Ctrl Pts',(-0.788671222413612,0.738083066750512,
0.12));
#5273=CARTESIAN_POINT('Ctrl Pts',(-0.807540237001567,0.715586030006559,
0.));
#5274=CARTESIAN_POINT('Ctrl Pts',(-0.807540237001567,0.715586030006559,
0.12));
#5275=CARTESIAN_POINT('Ctrl Pts',(-0.825780081176955,0.692596598957924,
0.));
#5276=CARTESIAN_POINT('Ctrl Pts',(-0.825780081176955,0.692596598957924,
0.12));
#5277=CARTESIAN_POINT('Ctrl Pts',(-0.843374934437182,0.669137170123487,
0.));
#5278=CARTESIAN_POINT('Ctrl Pts',(-0.843374934437182,0.669137170123487,
0.12));
#5279=CARTESIAN_POINT('Ctrl Pts',(-0.860309667736862,0.645230105164959,
0.));
#5280=CARTESIAN_POINT('Ctrl Pts',(-0.860309667736862,0.645230105164959,
0.12));
#5281=CARTESIAN_POINT('Ctrl Pts',(-0.876570783334186,0.620895981731371,
0.));
#5282=CARTESIAN_POINT('Ctrl Pts',(-0.876570783334186,0.620895981731371,
0.12));
#5283=CARTESIAN_POINT('Ctrl Pts',(-0.892147344046454,0.596151853069194,
0.));
#5284=CARTESIAN_POINT('Ctrl Pts',(-0.892147344046454,0.596151853069194,
0.12));
#5285=CARTESIAN_POINT('Ctrl Pts',(-0.90703203930424,0.571009280629087,0.));
#5286=CARTESIAN_POINT('Ctrl Pts',(-0.90703203930424,0.571009280629087,0.12));
#5287=CARTESIAN_POINT('Ctrl Pts',(-0.921220578942929,0.545475192012713,
0.));
#5288=CARTESIAN_POINT('Ctrl Pts',(-0.921220578942929,0.545475192012713,
0.12));
#5289=CARTESIAN_POINT('Ctrl Pts',(-0.932012813071653,0.524737521565861,
0.));
#5290=CARTESIAN_POINT('Ctrl Pts',(-0.932012813071653,0.524737521565861,
0.12));
#5291=CARTESIAN_POINT('Ctrl Pts',(-0.939792491219411,0.509010207622601,
0.));
#5292=CARTESIAN_POINT('Ctrl Pts',(-0.939792491219411,0.509010207622601,
0.12));
#5293=CARTESIAN_POINT('Ctrl Pts',(-0.944839172149305,0.498447974675534,
0.));
#5294=CARTESIAN_POINT('Ctrl Pts',(-0.944839172149305,0.498447974675534,
0.12));
#5295=CARTESIAN_POINT('Ctrl Pts',(-0.94732756983434,0.493147518935017,0.));
#5296=CARTESIAN_POINT('Ctrl Pts',(-0.94732756983434,0.493147518935017,0.12));
#5297=CARTESIAN_POINT('Ctrl Pts',(-0.8680312528477,-0.633495422775274,0.12));
#5298=CARTESIAN_POINT('Ctrl Pts',(-0.866468860926997,-0.635830722731769,
0.12));
#5299=CARTESIAN_POINT('Ctrl Pts',(-0.861627881960007,-0.64301558066062,
0.12));
#5300=CARTESIAN_POINT('Ctrl Pts',(-0.853391883864834,-0.654977418032855,
0.12));
#5301=CARTESIAN_POINT('Ctrl Pts',(-0.841545334406876,-0.671576597784011,
0.12));
#5302=CARTESIAN_POINT('Ctrl Pts',(-0.82578008117756,-0.69259659895799,0.12));
#5303=CARTESIAN_POINT('Ctrl Pts',(-0.807540237001814,-0.715586030006588,
0.12));
#5304=CARTESIAN_POINT('Ctrl Pts',(-0.788671222413511,-0.738083066750504,
0.12));
#5305=CARTESIAN_POINT('Ctrl Pts',(-0.769188516988648,-0.760067206050057,
0.12));
#5306=CARTESIAN_POINT('Ctrl Pts',(-0.749106566399864,-0.781521126617586,
0.12));
#5307=CARTESIAN_POINT('Ctrl Pts',(-0.728439343631846,-0.802429621210541,
0.12));
#5308=CARTESIAN_POINT('Ctrl Pts',(-0.707200722570354,-0.822778881439107,
0.12));
#5309=CARTESIAN_POINT('Ctrl Pts',(-0.685404899341998,-0.84255569314248,
0.12));
#5310=CARTESIAN_POINT('Ctrl Pts',(-0.663066855029994,-0.861746554484541,
0.12));
#5311=CARTESIAN_POINT('Ctrl Pts',(-0.640202597886525,-0.880337207900968,
0.12));
#5312=CARTESIAN_POINT('Ctrl Pts',(-0.61682888916888,-0.898313140761512,
0.12));
#5313=CARTESIAN_POINT('Ctrl Pts',(-0.592963069825771,-0.915659897318245,
0.12));
#5314=CARTESIAN_POINT('Ctrl Pts',(-0.568622860345861,-0.932363440835334,
0.12));
#5315=CARTESIAN_POINT('Ctrl Pts',(-0.543826140229843,-0.948410555212658,
0.12));
#5316=CARTESIAN_POINT('Ctrl Pts',(-0.518590849350175,-0.963789014835703,
0.12));
#5317=CARTESIAN_POINT('Ctrl Pts',(-0.492935086995462,-0.978487378620622,
0.12));
#5318=CARTESIAN_POINT('Ctrl Pts',(-0.466877166338143,-0.992494869297879,
0.12));
#5319=CARTESIAN_POINT('Ctrl Pts',(-0.440435680606148,-1.00580123015714,
0.12));
#5320=CARTESIAN_POINT('Ctrl Pts',(-0.413629579915119,-1.01839656305955,
0.12));
#5321=CARTESIAN_POINT('Ctrl Pts',(-0.386478184359591,-1.03027128325725,
0.12));
#5322=CARTESIAN_POINT('Ctrl Pts',(-0.359001120477101,-1.04141621492846,
0.12));
#5323=CARTESIAN_POINT('Ctrl Pts',(-0.331218276777395,-1.05182265203972,
0.12));
#5324=CARTESIAN_POINT('Ctrl Pts',(-0.30314975447047,-1.06148242804708,0.12));
#5325=CARTESIAN_POINT('Ctrl Pts',(-0.2748158132226,-1.07038799540312,0.12));
#5326=CARTESIAN_POINT('Ctrl Pts',(-0.246236848114779,-1.07853244619974,
0.12));
#5327=CARTESIAN_POINT('Ctrl Pts',(-0.217433396017985,-1.08590947721852,
0.12));
#5328=CARTESIAN_POINT('Ctrl Pts',(-0.188426134393584,-1.09251336987768,
0.12));
#5329=CARTESIAN_POINT('Ctrl Pts',(-0.159235881741527,-1.09833896639077,
0.12));
#5330=CARTESIAN_POINT('Ctrl Pts',(-0.129883601129733,-1.10338164243564,
0.12));
#5331=CARTESIAN_POINT('Ctrl Pts',(-0.100390386189668,-1.1076373045706,0.12));
#5332=CARTESIAN_POINT('Ctrl Pts',(-0.0707774336926613,-1.11110240713062,
0.12));
#5333=CARTESIAN_POINT('Ctrl Pts',(-0.0410660195909007,-1.11377396404697,
0.12));
#5334=CARTESIAN_POINT('Ctrl Pts',(-0.0112774747954127,-1.11564956182599,
0.12));
#5335=CARTESIAN_POINT('Ctrl Pts',(0.0185668417359402,-1.11672737500119,
0.12));
#5336=CARTESIAN_POINT('Ctrl Pts',(0.0484455558693415,-1.11700616793207,
0.12));
#5337=CARTESIAN_POINT('Ctrl Pts',(0.0783372821756426,-1.11648528736655,
0.12));
#5338=CARTESIAN_POINT('Ctrl Pts',(0.108220629786098,-1.11516465787405,0.12));
#5339=CARTESIAN_POINT('Ctrl Pts',(0.138074209040328,-1.1130447764894,0.12));
#5340=CARTESIAN_POINT('Ctrl Pts',(0.167876633777266,-1.11012670736124,0.12));
#5341=CARTESIAN_POINT('Ctrl Pts',(0.197606544321918,-1.10641207905813,0.12));
#5342=CARTESIAN_POINT('Ctrl Pts',(0.227242642150327,-1.10190308368776,0.12));
#5343=CARTESIAN_POINT('Ctrl Pts',(0.256763722532457,-1.09660247571268,0.12));
#5344=CARTESIAN_POINT('Ctrl Pts',(0.286148704656023,-1.09051357088032,0.12));
#5345=CARTESIAN_POINT('Ctrl Pts',(0.315376671295726,-1.08364024578391,0.12));
#5346=CARTESIAN_POINT('Ctrl Pts',(0.344426864523868,-1.07598693493533,0.12));
#5347=CARTESIAN_POINT('Ctrl Pts',(0.373278657560889,-1.06755862629372,0.12));
#5348=CARTESIAN_POINT('Ctrl Pts',(0.40191153059007,-1.05836085760139,0.12));
#5349=CARTESIAN_POINT('Ctrl Pts',(0.430305052465067,-1.04839971220046,0.12));
#5350=CARTESIAN_POINT('Ctrl Pts',(0.45843884125875,-1.03768181616585,0.12));
#5351=CARTESIAN_POINT('Ctrl Pts',(0.486292621102405,-1.02621433076827,0.12));
#5352=CARTESIAN_POINT('Ctrl Pts',(0.513846332693361,-1.01400494236352,0.12));
#5353=CARTESIAN_POINT('Ctrl Pts',(0.541080235433912,-1.00106185298107,0.12));
#5354=CARTESIAN_POINT('Ctrl Pts',(0.567974995595113,-0.987393771329312,
0.12));
#5355=CARTESIAN_POINT('Ctrl Pts',(0.594511824092215,-0.973009902467593,
0.12));
#5356=CARTESIAN_POINT('Ctrl Pts',(0.620672396673315,-0.957919944163756,
0.12));
#5357=CARTESIAN_POINT('Ctrl Pts',(0.646438641619482,-0.942134087249009,
0.12));
#5358=CARTESIAN_POINT('Ctrl Pts',(0.67179254905522,-0.925663015702513,0.12));
#5359=CARTESIAN_POINT('Ctrl Pts',(0.696716011515847,-0.908517905290565,
0.12));
#5360=CARTESIAN_POINT('Ctrl Pts',(0.721190552023322,-0.890710427237186,
0.12));
#5361=CARTESIAN_POINT('Ctrl Pts',(0.745197525414791,-0.872252731655685,
0.12));
#5362=CARTESIAN_POINT('Ctrl Pts',(0.768718652031186,-0.853157416735685,
0.12));
#5363=CARTESIAN_POINT('Ctrl Pts',(0.791736496209353,-0.833437500599933,
0.12));
#5364=CARTESIAN_POINT('Ctrl Pts',(0.814234876393174,-0.81310639575503,0.12));
#5365=CARTESIAN_POINT('Ctrl Pts',(0.836199528793963,-0.792177873864096,
0.12));
#5366=CARTESIAN_POINT('Ctrl Pts',(0.857617760934752,-0.770666069833932,
0.12));
#5367=CARTESIAN_POINT('Ctrl Pts',(0.878477242115376,-0.74858551944097,0.12));
#5368=CARTESIAN_POINT('Ctrl Pts',(0.898764943113291,-0.725951191437368,
0.12));
#5369=CARTESIAN_POINT('Ctrl Pts',(0.918466214618678,-0.70277851394702,0.12));
#5370=CARTESIAN_POINT('Ctrl Pts',(0.937563319582499,-0.679083423181946,
0.12));
#5371=CARTESIAN_POINT('Ctrl Pts',(0.956036026761672,-0.654882328595489,
0.12));
#5372=CARTESIAN_POINT('Ctrl Pts',(0.973864462863685,-0.630191986422907,
0.12));
#5373=CARTESIAN_POINT('Ctrl Pts',(0.991031566790864,-0.605029389584474,
0.12));
#5374=CARTESIAN_POINT('Ctrl Pts',(1.00752529081786,-0.579411667627393,0.12));
#5375=CARTESIAN_POINT('Ctrl Pts',(1.02334191285221,-0.553355942423953,0.12));
#5376=CARTESIAN_POINT('Ctrl Pts',(1.03848536635828,-0.526879343018338,0.12));
#5377=CARTESIAN_POINT('Ctrl Pts',(1.05296063073153,-0.499999257829972,0.12));
#5378=CARTESIAN_POINT('Ctrl Pts',(1.06676816041365,-0.472733545459157,0.12));
#5379=CARTESIAN_POINT('Ctrl Pts',(1.0798986829592,-0.44510073074649,0.12));
#5380=CARTESIAN_POINT('Ctrl Pts',(1.09232595504273,-0.417120282666841,0.12));
#5381=CARTESIAN_POINT('Ctrl Pts',(1.1040065500515,-0.388812610728411,0.12));
#5382=CARTESIAN_POINT('Ctrl Pts',(1.11489509573247,-0.360198442057814,0.12));
#5383=CARTESIAN_POINT('Ctrl Pts',(1.12495696400084,-0.331298301519,0.12));
#5384=CARTESIAN_POINT('Ctrl Pts',(1.13418071785862,-0.302131999517994,0.12));
#5385=CARTESIAN_POINT('Ctrl Pts',(1.14259364432097,-0.272718001214759,0.12));
#5386=CARTESIAN_POINT('Ctrl Pts',(1.15026681194464,-0.243073201156197,0.12));
#5387=CARTESIAN_POINT('Ctrl Pts',(1.15728135528338,-0.213214209193066,0.12));
#5388=CARTESIAN_POINT('Ctrl Pts',(1.16370031035361,-0.183158411923726,0.12));
#5389=CARTESIAN_POINT('Ctrl Pts',(1.1695394362355,-0.152925093725504,0.12));
#5390=CARTESIAN_POINT('Ctrl Pts',(1.17473573615846,-0.1225365994934,0.12));
#5391=CARTESIAN_POINT('Ctrl Pts',(1.17912488557723,-0.0920192855934153,
0.12));
#5392=CARTESIAN_POINT('Ctrl Pts',(1.18249458653374,-0.0614026081204919,
0.12));
#5393=CARTESIAN_POINT('Ctrl Pts',(1.18463081328693,-0.0307183863950716,
0.12));
#5394=CARTESIAN_POINT('Ctrl Pts',(1.18536679600018,3.34053531364509E-15,
0.12));
#5395=CARTESIAN_POINT('Ctrl Pts',(1.18463081328694,0.0307183863950759,0.12));
#5396=CARTESIAN_POINT('Ctrl Pts',(1.18249458653375,0.0614026081204918,0.12));
#5397=CARTESIAN_POINT('Ctrl Pts',(1.17912488557725,0.0920192855934129,0.12));
#5398=CARTESIAN_POINT('Ctrl Pts',(1.17473573615847,0.122536599493401,0.12));
#5399=CARTESIAN_POINT('Ctrl Pts',(1.1695394362355,0.152925093725509,0.12));
#5400=CARTESIAN_POINT('Ctrl Pts',(1.1637003103536,0.183158411923732,0.12));
#5401=CARTESIAN_POINT('Ctrl Pts',(1.15728135528336,0.21321420919307,0.12));
#5402=CARTESIAN_POINT('Ctrl Pts',(1.15026681194462,0.243073201156195,0.12));
#5403=CARTESIAN_POINT('Ctrl Pts',(1.14259364432096,0.272718001214758,0.12));
#5404=CARTESIAN_POINT('Ctrl Pts',(1.13418071785862,0.302131999517997,0.12));
#5405=CARTESIAN_POINT('Ctrl Pts',(1.12495696400085,0.33129830151901,0.12));
#5406=CARTESIAN_POINT('Ctrl Pts',(1.11489509573248,0.36019844205783,0.12));
#5407=CARTESIAN_POINT('Ctrl Pts',(1.10400655005151,0.388812610728428,0.12));
#5408=CARTESIAN_POINT('Ctrl Pts',(1.09232595504274,0.417120282666858,0.12));
#5409=CARTESIAN_POINT('Ctrl Pts',(1.0798986829592,0.4451007307465,0.12));
#5410=CARTESIAN_POINT('Ctrl Pts',(1.06676816041364,0.472733545459153,0.12));
#5411=CARTESIAN_POINT('Ctrl Pts',(1.05296063073151,0.499999257829953,0.12));
#5412=CARTESIAN_POINT('Ctrl Pts',(1.03848536635825,0.526879343018311,0.12));
#5413=CARTESIAN_POINT('Ctrl Pts',(1.02334191285218,0.553355942423933,0.12));
#5414=CARTESIAN_POINT('Ctrl Pts',(1.00752529081784,0.579411667627389,0.12));
#5415=CARTESIAN_POINT('Ctrl Pts',(0.991031566790874,0.605029389584491,0.12));
#5416=CARTESIAN_POINT('Ctrl Pts',(0.973864462863717,0.630191986422942,0.12));
#5417=CARTESIAN_POINT('Ctrl Pts',(0.956036026761713,0.654882328595531,0.12));
#5418=CARTESIAN_POINT('Ctrl Pts',(0.93756331958253,0.67908342318198,0.12));
#5419=CARTESIAN_POINT('Ctrl Pts',(0.918466214618686,0.702778513947035,0.12));
#5420=CARTESIAN_POINT('Ctrl Pts',(0.898764943113273,0.725951191437361,0.12));
#5421=CARTESIAN_POINT('Ctrl Pts',(0.87847724211534,0.748585519440939,0.12));
#5422=CARTESIAN_POINT('Ctrl Pts',(0.857617760934708,0.770666069833888,0.12));
#5423=CARTESIAN_POINT('Ctrl Pts',(0.836199528793927,0.792177873864058,0.12));
#5424=CARTESIAN_POINT('Ctrl Pts',(0.814234876393157,0.813106395755015,0.12));
#5425=CARTESIAN_POINT('Ctrl Pts',(0.79173649620936,0.833437500599952,0.12));
#5426=CARTESIAN_POINT('Ctrl Pts',(0.768718652031217,0.853157416735736,0.12));
#5427=CARTESIAN_POINT('Ctrl Pts',(0.745197525414833,0.872252731655753,0.12));
#5428=CARTESIAN_POINT('Ctrl Pts',(0.721190552023354,0.890710427237242,0.12));
#5429=CARTESIAN_POINT('Ctrl Pts',(0.696716011515856,0.908517905290589,0.12));
#5430=CARTESIAN_POINT('Ctrl Pts',(0.671792549055205,0.9256630157025,0.12));
#5431=CARTESIAN_POINT('Ctrl Pts',(0.64643864161945,0.942134087248967,0.12));
#5432=CARTESIAN_POINT('Ctrl Pts',(0.620672396673277,0.95791994416371,0.12));
#5433=CARTESIAN_POINT('Ctrl Pts',(0.594511824092183,0.973009902467561,0.12));
#5434=CARTESIAN_POINT('Ctrl Pts',(0.567974995595098,0.987393771329304,0.12));
#5435=CARTESIAN_POINT('Ctrl Pts',(0.541080235433915,1.00106185298108,0.12));
#5436=CARTESIAN_POINT('Ctrl Pts',(0.513846332693379,1.01400494236354,0.12));
#5437=CARTESIAN_POINT('Ctrl Pts',(0.486292621102429,1.02621433076829,0.12));
#5438=CARTESIAN_POINT('Ctrl Pts',(0.458438841258773,1.03768181616586,0.12));
#5439=CARTESIAN_POINT('Ctrl Pts',(0.430305052465076,1.04839971220046,0.12));
#5440=CARTESIAN_POINT('Ctrl Pts',(0.401911530590058,1.05836085760139,0.12));
#5441=CARTESIAN_POINT('Ctrl Pts',(0.373278657560858,1.06755862629372,0.12));
#5442=CARTESIAN_POINT('Ctrl Pts',(0.344426864523825,1.07598693493533,0.12));
#5443=CARTESIAN_POINT('Ctrl Pts',(0.315376671295687,1.08364024578392,0.12));
#5444=CARTESIAN_POINT('Ctrl Pts',(0.286148704656,1.09051357088032,0.12));
#5445=CARTESIAN_POINT('Ctrl Pts',(0.256763722532462,1.09660247571268,0.12));
#5446=CARTESIAN_POINT('Ctrl Pts',(0.22724264215036,1.10190308368774,0.12));
#5447=CARTESIAN_POINT('Ctrl Pts',(0.197606544321966,1.10641207905811,0.12));
#5448=CARTESIAN_POINT('Ctrl Pts',(0.167876633777302,1.11012670736122,0.12));
#5449=CARTESIAN_POINT('Ctrl Pts',(0.138074209040338,1.11304477648939,0.12));
#5450=CARTESIAN_POINT('Ctrl Pts',(0.108220629786082,1.11516465787406,0.12));
#5451=CARTESIAN_POINT('Ctrl Pts',(0.0783372821756164,1.11648528736656,0.12));
#5452=CARTESIAN_POINT('Ctrl Pts',(0.0484455558693182,1.11700616793208,0.12));
#5453=CARTESIAN_POINT('Ctrl Pts',(0.0185668417359279,1.1167273750012,0.12));
#5454=CARTESIAN_POINT('Ctrl Pts',(-0.011277474795416,1.11564956182599,0.12));
#5455=CARTESIAN_POINT('Ctrl Pts',(-0.041066019590905,1.11377396404697,0.12));
#5456=CARTESIAN_POINT('Ctrl Pts',(-0.0707774336926752,1.11110240713063,
0.12));
#5457=CARTESIAN_POINT('Ctrl Pts',(-0.100390386189687,1.10763730457062,0.12));
#5458=CARTESIAN_POINT('Ctrl Pts',(-0.129883601129753,1.10338164243566,0.12));
#5459=CARTESIAN_POINT('Ctrl Pts',(-0.159235881741536,1.09833896639078,0.12));
#5460=CARTESIAN_POINT('Ctrl Pts',(-0.188426134393585,1.09251336987768,0.12));
#5461=CARTESIAN_POINT('Ctrl Pts',(-0.217433396017983,1.08590947721851,0.12));
#5462=CARTESIAN_POINT('Ctrl Pts',(-0.246236848114778,1.07853244619972,0.12));
#5463=CARTESIAN_POINT('Ctrl Pts',(-0.274815813222603,1.07038799540312,0.12));
#5464=CARTESIAN_POINT('Ctrl Pts',(-0.303149754470475,1.06148242804708,0.12));
#5465=CARTESIAN_POINT('Ctrl Pts',(-0.3312182767774,1.05182265203972,0.12));
#5466=CARTESIAN_POINT('Ctrl Pts',(-0.359001120477101,1.04141621492845,0.12));
#5467=CARTESIAN_POINT('Ctrl Pts',(-0.386478184359588,1.03027128325725,0.12));
#5468=CARTESIAN_POINT('Ctrl Pts',(-0.413629579915113,1.01839656305955,0.12));
#5469=CARTESIAN_POINT('Ctrl Pts',(-0.440435680606144,1.00580123015714,0.12));
#5470=CARTESIAN_POINT('Ctrl Pts',(-0.466877166338154,0.992494869297873,
0.12));
#5471=CARTESIAN_POINT('Ctrl Pts',(-0.492935086995497,0.97848737862061,0.12));
#5472=CARTESIAN_POINT('Ctrl Pts',(-0.518590849350232,0.963789014835687,
0.12));
#5473=CARTESIAN_POINT('Ctrl Pts',(-0.5438261402299,0.948410555212641,0.12));
#5474=CARTESIAN_POINT('Ctrl Pts',(-0.568622860345892,0.932363440835325,
0.12));
#5475=CARTESIAN_POINT('Ctrl Pts',(-0.592963069825743,0.91565989731825,0.12));
#5476=CARTESIAN_POINT('Ctrl Pts',(-0.616828889168791,0.898313140761531,
0.12));
#5477=CARTESIAN_POINT('Ctrl Pts',(-0.64020259788639,0.880337207900991,0.12));
#5478=CARTESIAN_POINT('Ctrl Pts',(-0.663066855029865,0.861746554484547,
0.12));
#5479=CARTESIAN_POINT('Ctrl Pts',(-0.685404899341948,0.842555693142475,
0.12));
#5480=CARTESIAN_POINT('Ctrl Pts',(-0.707200722570447,0.822778881439102,
0.12));
#5481=CARTESIAN_POINT('Ctrl Pts',(-0.728439343632102,0.802429621210551,
0.12));
#5482=CARTESIAN_POINT('Ctrl Pts',(-0.749106566400217,0.781521126617609,
0.12));
#5483=CARTESIAN_POINT('Ctrl Pts',(-0.76918851698896,0.760067206050081,0.12));
#5484=CARTESIAN_POINT('Ctrl Pts',(-0.788671222413612,0.738083066750512,
0.12));
#5485=CARTESIAN_POINT('Ctrl Pts',(-0.807540237001567,0.715586030006559,
0.12));
#5486=CARTESIAN_POINT('Ctrl Pts',(-0.825780081176955,0.692596598957924,
0.12));
#5487=CARTESIAN_POINT('Ctrl Pts',(-0.841545334406124,0.671576597783911,
0.12));
#5488=CARTESIAN_POINT('Ctrl Pts',(-0.85339188386416,0.654977418032737,0.12));
#5489=CARTESIAN_POINT('Ctrl Pts',(-0.861627881959507,0.643015580660492,
0.12));
#5490=CARTESIAN_POINT('Ctrl Pts',(-0.866468860926645,0.635830722731627,
0.12));
#5491=CARTESIAN_POINT('Ctrl Pts',(-0.868031252847412,0.633495422775111,
0.12));
#5492=CARTESIAN_POINT('Origin',(0.11901961308292,6.21724893790088E-15,0.12));
#5515=UNCERTAINTY_MEASURE_WITH_UNIT(LENGTH_MEASURE(0.001),#5536,
'DISTANCE_ACCURACY_VALUE',
'Maximum model space distance between geometric entities at asserted c
onnectivities');
#5516=UNCERTAINTY_MEASURE_WITH_UNIT(LENGTH_MEASURE(0.001),#5536,
'DISTANCE_ACCURACY_VALUE',
'Maximum model space distance between geometric entities at asserted c
onnectivities');
#5534=(
GEOMETRIC_REPRESENTATION_CONTEXT(3)
GLOBAL_UNCERTAINTY_ASSIGNED_CONTEXT((#5515))
GLOBAL_UNIT_ASSIGNED_CONTEXT((#5536,#5538,#5539))
REPRESENTATION_CONTEXT('','3D')
);
#5535=(
GEOMETRIC_REPRESENTATION_CONTEXT(3)
GLOBAL_UNCERTAINTY_ASSIGNED_CONTEXT((#5516))
GLOBAL_UNIT_ASSIGNED_CONTEXT((#5536,#5538,#5539))
REPRESENTATION_CONTEXT('','3D')
);
#5536=(
LENGTH_UNIT()
NAMED_UNIT(*)
SI_UNIT(.CENTI.,.METRE.)
);
#5538=(
NAMED_UNIT(*)
PLANE_ANGLE_UNIT()
SI_UNIT($,.RADIAN.)
);
#5539=(
NAMED_UNIT(*)
SI_UNIT($,.STERADIAN.)
SOLID_ANGLE_UNIT()
);
#5557=SHAPE_DEFINITION_REPRESENTATION(#5595,#5618);
#5595=PRODUCT_DEFINITION_SHAPE('',$,#5637);
#5618=SHAPE_REPRESENTATION('',(#2844),#5534);
#5619=PRODUCT_DEFINITION_CONTEXT('part definition',#5675,'design');
#5637=PRODUCT_DEFINITION('Installed retaining ring',
'Installed retaining ring',#5655,#5619);
#5655=PRODUCT_DEFINITION_FORMATION('',$,#5694);
#5675=APPLICATION_CONTEXT(
'Core Data for Automotive Mechanical Design Process');
#5676=PRODUCT_CONTEXT('part definition',#5675,'mechanical');
#5694=PRODUCT('Installed retaining ring','Installed retaining ring',
'Installed retaining ring',(#5676));
#5772=COLOUR_RGB('Off White',0.89,0.88,0.83);
#5773=FILL_AREA_STYLE_COLOUR('',#5772);
#5774=FILL_AREA_STYLE('',(#5773));
#5775=SURFACE_STYLE_FILL_AREA(#5774);
#5776=SURFACE_SIDE_STYLE('',(#5775));
#5777=SURFACE_STYLE_USAGE(.BOTH.,#5776);
#5778=PRESENTATION_STYLE_ASSIGNMENT((#5777));
ENDSEC;
END-ISO-10303-21;
